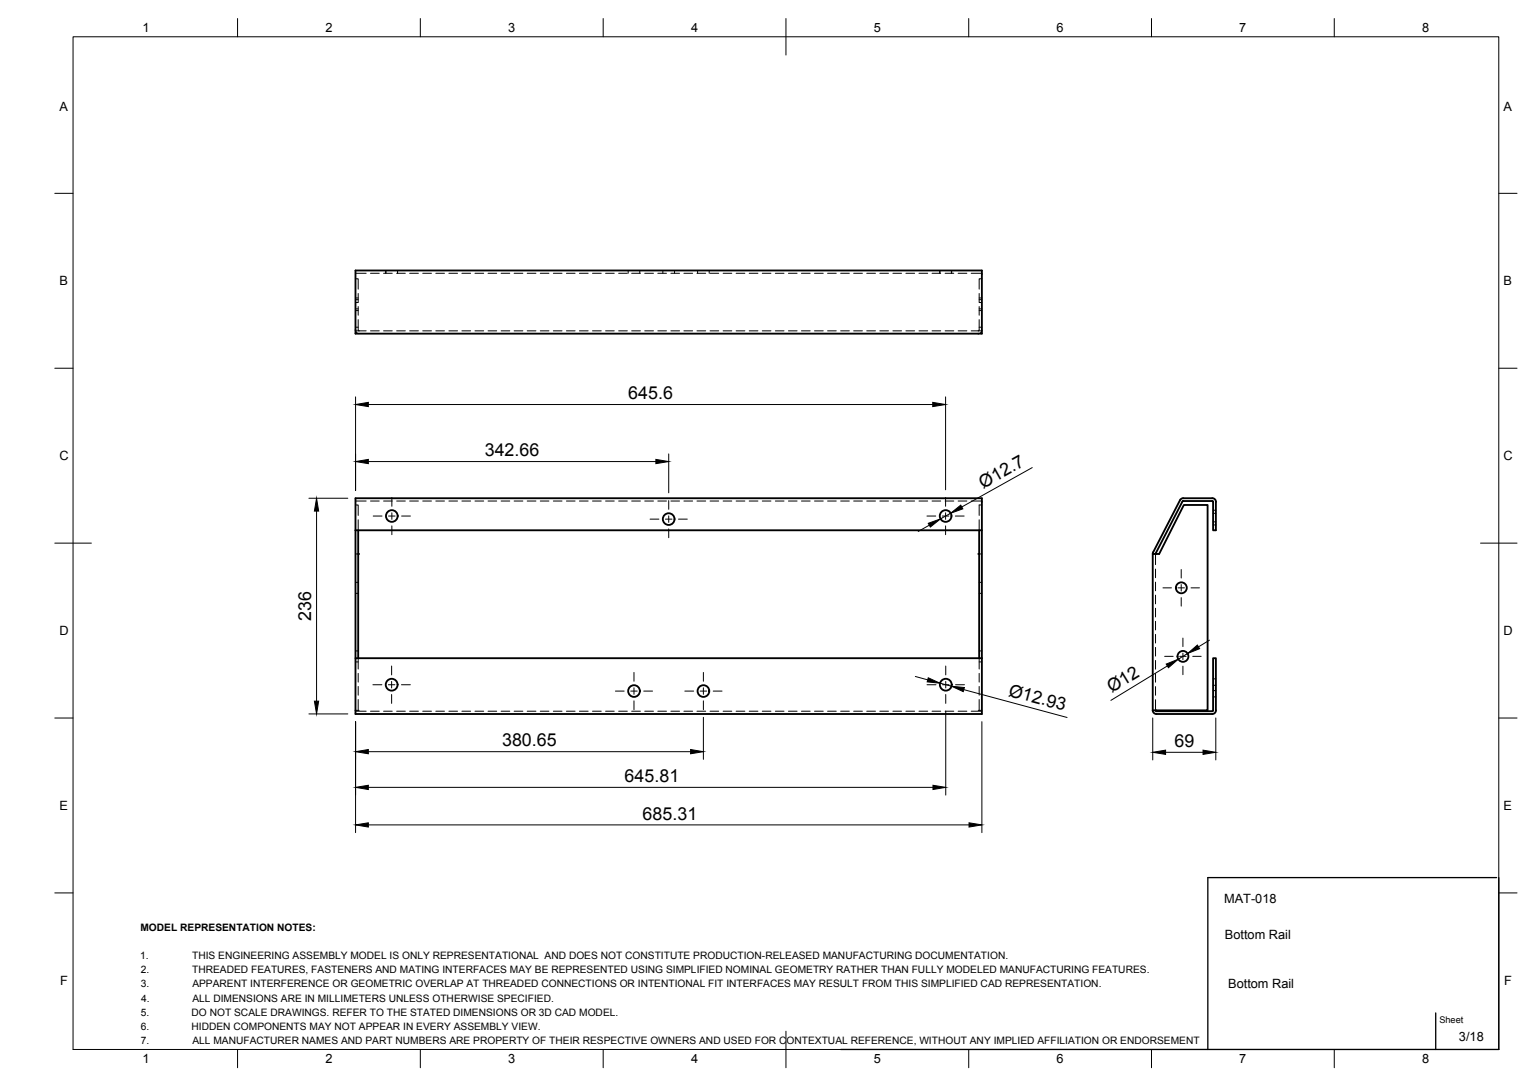
ISO-10303-21;
HEADER;
/* Generated by software containing ST-Developer
 * from STEP Tools, Inc. (www.steptools.com) 
 */

FILE_DESCRIPTION(
/* description */ ('STEP AP214'),
/* implementation_level */ '2;1');

FILE_NAME(
/* name */ 'Bottom Rail.step',
/* time_stamp */ '2026-11-14T06:16:09-08:00',
/* author */ (''),
/* organization */ (''),
/* preprocessor_version */ 'ST-DEVELOPER v20.2',
/* originating_system */ 'Autodesk Translation Framework v15.17.0.0',
/* authorisation */ '');

FILE_SCHEMA (('AUTOMOTIVE_DESIGN { 1 0 10303 214 3 1 1 }'));
ENDSEC;

DATA;
#10=MECHANICAL_DESIGN_GEOMETRIC_PRESENTATION_REPRESENTATION('',(#347),#18006);
#315=SHAPE_REPRESENTATION_RELATIONSHIP('SRR','None',#18071,#331);
#331=ADVANCED_BREP_SHAPE_REPRESENTATION('',(#363),#17988);
#347=STYLED_ITEM('',(#18170),#363);
#363=MANIFOLD_SOLID_BREP('Body1',#9556);
#379=FACE_BOUND('',#1453,.T.);
#380=FACE_BOUND('',#1454,.T.);
#381=FACE_BOUND('',#1455,.T.);
#382=FACE_BOUND('',#1456,.T.);
#383=FACE_BOUND('',#1459,.T.);
#384=FACE_BOUND('',#1460,.T.);
#385=FACE_BOUND('',#1461,.T.);
#386=FACE_BOUND('',#1462,.T.);
#387=FACE_BOUND('',#1472,.T.);
#388=FACE_BOUND('',#1473,.T.);
#389=FACE_BOUND('',#1474,.T.);
#390=FACE_BOUND('',#1477,.T.);
#391=FACE_BOUND('',#1478,.T.);
#392=FACE_BOUND('',#1479,.T.);
#393=FACE_BOUND('',#1497,.T.);
#394=FACE_BOUND('',#1498,.T.);
#395=FACE_BOUND('',#1500,.T.);
#396=FACE_BOUND('',#1501,.T.);
#397=FACE_BOUND('',#1512,.T.);
#398=FACE_BOUND('',#1513,.T.);
#399=FACE_BOUND('',#1515,.T.);
#400=FACE_BOUND('',#1516,.T.);
#502=PLANE('',#9784);
#503=PLANE('',#9786);
#504=PLANE('',#9788);
#505=PLANE('',#9789);
#506=PLANE('',#9790);
#507=PLANE('',#9792);
#508=PLANE('',#9794);
#509=PLANE('',#9797);
#510=PLANE('',#9798);
#511=PLANE('',#9801);
#512=PLANE('',#9802);
#513=PLANE('',#9805);
#514=PLANE('',#9806);
#515=PLANE('',#9809);
#516=PLANE('',#9810);
#517=PLANE('',#9813);
#518=PLANE('',#9816);
#519=PLANE('',#9817);
#520=PLANE('',#9820);
#521=PLANE('',#9821);
#522=PLANE('',#9824);
#523=PLANE('',#9827);
#524=PLANE('',#9828);
#525=PLANE('',#9831);
#526=PLANE('',#9832);
#527=PLANE('',#9833);
#528=PLANE('',#9834);
#529=PLANE('',#9836);
#530=PLANE('',#9839);
#531=PLANE('',#9841);
#532=PLANE('',#9843);
#533=PLANE('',#9844);
#534=PLANE('',#9845);
#535=PLANE('',#9847);
#536=PLANE('',#9849);
#537=PLANE('',#9852);
#538=PLANE('',#9854);
#539=PLANE('',#9855);
#540=PLANE('',#9856);
#541=PLANE('',#9859);
#542=PLANE('',#9864);
#543=PLANE('',#9865);
#544=PLANE('',#9866);
#545=PLANE('',#9867);
#546=PLANE('',#9868);
#547=PLANE('',#9869);
#548=PLANE('',#9870);
#549=PLANE('',#9871);
#550=PLANE('',#9874);
#551=PLANE('',#9879);
#552=PLANE('',#9880);
#553=PLANE('',#9881);
#554=PLANE('',#9882);
#555=PLANE('',#9883);
#556=PLANE('',#9884);
#557=PLANE('',#9885);
#841=FACE_OUTER_BOUND('',#1417,.T.);
#842=FACE_OUTER_BOUND('',#1418,.T.);
#843=FACE_OUTER_BOUND('',#1419,.T.);
#844=FACE_OUTER_BOUND('',#1420,.T.);
#845=FACE_OUTER_BOUND('',#1421,.T.);
#846=FACE_OUTER_BOUND('',#1422,.T.);
#847=FACE_OUTER_BOUND('',#1423,.T.);
#848=FACE_OUTER_BOUND('',#1424,.T.);
#849=FACE_OUTER_BOUND('',#1425,.T.);
#850=FACE_OUTER_BOUND('',#1426,.T.);
#851=FACE_OUTER_BOUND('',#1427,.T.);
#852=FACE_OUTER_BOUND('',#1428,.T.);
#853=FACE_OUTER_BOUND('',#1429,.T.);
#854=FACE_OUTER_BOUND('',#1430,.T.);
#855=FACE_OUTER_BOUND('',#1431,.T.);
#856=FACE_OUTER_BOUND('',#1432,.T.);
#857=FACE_OUTER_BOUND('',#1433,.T.);
#858=FACE_OUTER_BOUND('',#1434,.T.);
#859=FACE_OUTER_BOUND('',#1435,.T.);
#860=FACE_OUTER_BOUND('',#1436,.T.);
#861=FACE_OUTER_BOUND('',#1437,.T.);
#862=FACE_OUTER_BOUND('',#1438,.T.);
#863=FACE_OUTER_BOUND('',#1439,.T.);
#864=FACE_OUTER_BOUND('',#1440,.T.);
#865=FACE_OUTER_BOUND('',#1441,.T.);
#866=FACE_OUTER_BOUND('',#1442,.T.);
#867=FACE_OUTER_BOUND('',#1443,.T.);
#868=FACE_OUTER_BOUND('',#1444,.T.);
#869=FACE_OUTER_BOUND('',#1445,.T.);
#870=FACE_OUTER_BOUND('',#1446,.T.);
#871=FACE_OUTER_BOUND('',#1447,.T.);
#872=FACE_OUTER_BOUND('',#1448,.T.);
#873=FACE_OUTER_BOUND('',#1449,.T.);
#874=FACE_OUTER_BOUND('',#1450,.T.);
#875=FACE_OUTER_BOUND('',#1451,.T.);
#876=FACE_OUTER_BOUND('',#1452,.T.);
#877=FACE_OUTER_BOUND('',#1457,.T.);
#878=FACE_OUTER_BOUND('',#1458,.T.);
#879=FACE_OUTER_BOUND('',#1463,.T.);
#880=FACE_OUTER_BOUND('',#1464,.T.);
#881=FACE_OUTER_BOUND('',#1465,.T.);
#882=FACE_OUTER_BOUND('',#1466,.T.);
#883=FACE_OUTER_BOUND('',#1467,.T.);
#884=FACE_OUTER_BOUND('',#1468,.T.);
#885=FACE_OUTER_BOUND('',#1469,.T.);
#886=FACE_OUTER_BOUND('',#1470,.T.);
#887=FACE_OUTER_BOUND('',#1471,.T.);
#888=FACE_OUTER_BOUND('',#1475,.T.);
#889=FACE_OUTER_BOUND('',#1476,.T.);
#890=FACE_OUTER_BOUND('',#1480,.T.);
#891=FACE_OUTER_BOUND('',#1481,.T.);
#892=FACE_OUTER_BOUND('',#1482,.T.);
#893=FACE_OUTER_BOUND('',#1483,.T.);
#894=FACE_OUTER_BOUND('',#1484,.T.);
#895=FACE_OUTER_BOUND('',#1485,.T.);
#896=FACE_OUTER_BOUND('',#1486,.T.);
#897=FACE_OUTER_BOUND('',#1487,.T.);
#898=FACE_OUTER_BOUND('',#1488,.T.);
#899=FACE_OUTER_BOUND('',#1489,.T.);
#900=FACE_OUTER_BOUND('',#1490,.T.);
#901=FACE_OUTER_BOUND('',#1491,.T.);
#902=FACE_OUTER_BOUND('',#1492,.T.);
#903=FACE_OUTER_BOUND('',#1493,.T.);
#904=FACE_OUTER_BOUND('',#1494,.T.);
#905=FACE_OUTER_BOUND('',#1495,.T.);
#906=FACE_OUTER_BOUND('',#1496,.T.);
#907=FACE_OUTER_BOUND('',#1499,.T.);
#908=FACE_OUTER_BOUND('',#1502,.T.);
#909=FACE_OUTER_BOUND('',#1503,.T.);
#910=FACE_OUTER_BOUND('',#1504,.T.);
#911=FACE_OUTER_BOUND('',#1505,.T.);
#912=FACE_OUTER_BOUND('',#1506,.T.);
#913=FACE_OUTER_BOUND('',#1507,.T.);
#914=FACE_OUTER_BOUND('',#1508,.T.);
#915=FACE_OUTER_BOUND('',#1509,.T.);
#916=FACE_OUTER_BOUND('',#1510,.T.);
#917=FACE_OUTER_BOUND('',#1511,.T.);
#918=FACE_OUTER_BOUND('',#1514,.T.);
#919=FACE_OUTER_BOUND('',#1517,.T.);
#920=FACE_OUTER_BOUND('',#1518,.T.);
#921=FACE_OUTER_BOUND('',#1519,.T.);
#1417=EDGE_LOOP('',(#6152,#6153,#6154,#6155));
#1418=EDGE_LOOP('',(#6156,#6157,#6158,#6159));
#1419=EDGE_LOOP('',(#6160,#6161,#6162,#6163));
#1420=EDGE_LOOP('',(#6164,#6165,#6166,#6167));
#1421=EDGE_LOOP('',(#6168,#6169,#6170,#6171));
#1422=EDGE_LOOP('',(#6172,#6173,#6174,#6175));
#1423=EDGE_LOOP('',(#6176,#6177,#6178,#6179));
#1424=EDGE_LOOP('',(#6180,#6181,#6182,#6183));
#1425=EDGE_LOOP('',(#6184,#6185,#6186,#6187));
#1426=EDGE_LOOP('',(#6188,#6189,#6190,#6191));
#1427=EDGE_LOOP('',(#6192,#6193,#6194,#6195));
#1428=EDGE_LOOP('',(#6196,#6197,#6198,#6199));
#1429=EDGE_LOOP('',(#6200,#6201,#6202,#6203));
#1430=EDGE_LOOP('',(#6204,#6205,#6206,#6207));
#1431=EDGE_LOOP('',(#6208,#6209,#6210,#6211));
#1432=EDGE_LOOP('',(#6212,#6213,#6214,#6215));
#1433=EDGE_LOOP('',(#6216,#6217,#6218,#6219));
#1434=EDGE_LOOP('',(#6220,#6221,#6222,#6223));
#1435=EDGE_LOOP('',(#6224,#6225,#6226,#6227));
#1436=EDGE_LOOP('',(#6228,#6229,#6230,#6231));
#1437=EDGE_LOOP('',(#6232,#6233,#6234,#6235));
#1438=EDGE_LOOP('',(#6236,#6237,#6238,#6239));
#1439=EDGE_LOOP('',(#6240,#6241,#6242,#6243));
#1440=EDGE_LOOP('',(#6244,#6245,#6246,#6247));
#1441=EDGE_LOOP('',(#6248,#6249,#6250,#6251));
#1442=EDGE_LOOP('',(#6252,#6253,#6254,#6255));
#1443=EDGE_LOOP('',(#6256,#6257,#6258,#6259));
#1444=EDGE_LOOP('',(#6260,#6261,#6262,#6263));
#1445=EDGE_LOOP('',(#6264,#6265,#6266,#6267));
#1446=EDGE_LOOP('',(#6268,#6269,#6270,#6271));
#1447=EDGE_LOOP('',(#6272,#6273,#6274,#6275));
#1448=EDGE_LOOP('',(#6276,#6277,#6278,#6279));
#1449=EDGE_LOOP('',(#6280,#6281,#6282,#6283));
#1450=EDGE_LOOP('',(#6284,#6285,#6286,#6287));
#1451=EDGE_LOOP('',(#6288,#6289,#6290,#6291));
#1452=EDGE_LOOP('',(#6292,#6293,#6294,#6295));
#1453=EDGE_LOOP('',(#6296));
#1454=EDGE_LOOP('',(#6297));
#1455=EDGE_LOOP('',(#6298));
#1456=EDGE_LOOP('',(#6299));
#1457=EDGE_LOOP('',(#6300,#6301,#6302,#6303));
#1458=EDGE_LOOP('',(#6304,#6305,#6306,#6307));
#1459=EDGE_LOOP('',(#6308));
#1460=EDGE_LOOP('',(#6309));
#1461=EDGE_LOOP('',(#6310));
#1462=EDGE_LOOP('',(#6311));
#1463=EDGE_LOOP('',(#6312,#6313,#6314,#6315));
#1464=EDGE_LOOP('',(#6316,#6317,#6318,#6319));
#1465=EDGE_LOOP('',(#6320,#6321,#6322,#6323,#6324,#6325));
#1466=EDGE_LOOP('',(#6326,#6327,#6328,#6329,#6330,#6331));
#1467=EDGE_LOOP('',(#6332,#6333,#6334,#6335));
#1468=EDGE_LOOP('',(#6336,#6337,#6338,#6339));
#1469=EDGE_LOOP('',(#6340,#6341,#6342,#6343));
#1470=EDGE_LOOP('',(#6344,#6345,#6346,#6347));
#1471=EDGE_LOOP('',(#6348,#6349,#6350,#6351));
#1472=EDGE_LOOP('',(#6352));
#1473=EDGE_LOOP('',(#6353));
#1474=EDGE_LOOP('',(#6354));
#1475=EDGE_LOOP('',(#6355,#6356,#6357,#6358));
#1476=EDGE_LOOP('',(#6359,#6360,#6361,#6362));
#1477=EDGE_LOOP('',(#6363));
#1478=EDGE_LOOP('',(#6364));
#1479=EDGE_LOOP('',(#6365));
#1480=EDGE_LOOP('',(#6366,#6367,#6368,#6369));
#1481=EDGE_LOOP('',(#6370,#6371,#6372,#6373));
#1482=EDGE_LOOP('',(#6374,#6375,#6376,#6377));
#1483=EDGE_LOOP('',(#6378,#6379,#6380,#6381));
#1484=EDGE_LOOP('',(#6382,#6383,#6384,#6385,#6386,#6387,#6388,#6389));
#1485=EDGE_LOOP('',(#6390,#6391,#6392,#6393,#6394,#6395,#6396,#6397));
#1486=EDGE_LOOP('',(#6398,#6399,#6400,#6401));
#1487=EDGE_LOOP('',(#6402,#6403,#6404,#6405));
#1488=EDGE_LOOP('',(#6406,#6407,#6408,#6409));
#1489=EDGE_LOOP('',(#6410,#6411,#6412,#6413));
#1490=EDGE_LOOP('',(#6414,#6415,#6416,#6417));
#1491=EDGE_LOOP('',(#6418,#6419,#6420,#6421));
#1492=EDGE_LOOP('',(#6422,#6423,#6424,#6425,#6426,#6427));
#1493=EDGE_LOOP('',(#6428,#6429,#6430,#6431));
#1494=EDGE_LOOP('',(#6432,#6433,#6434,#6435));
#1495=EDGE_LOOP('',(#6436,#6437,#6438,#6439));
#1496=EDGE_LOOP('',(#6440,#6441,#6442,#6443,#6444,#6445));
#1497=EDGE_LOOP('',(#6446));
#1498=EDGE_LOOP('',(#6447));
#1499=EDGE_LOOP('',(#6448,#6449,#6450,#6451,#6452,#6453));
#1500=EDGE_LOOP('',(#6454));
#1501=EDGE_LOOP('',(#6455));
#1502=EDGE_LOOP('',(#6456,#6457,#6458,#6459));
#1503=EDGE_LOOP('',(#6460,#6461,#6462,#6463));
#1504=EDGE_LOOP('',(#6464,#6465,#6466,#6467));
#1505=EDGE_LOOP('',(#6468,#6469,#6470,#6471));
#1506=EDGE_LOOP('',(#6472,#6473,#6474,#6475));
#1507=EDGE_LOOP('',(#6476,#6477,#6478,#6479,#6480,#6481));
#1508=EDGE_LOOP('',(#6482,#6483,#6484,#6485));
#1509=EDGE_LOOP('',(#6486,#6487,#6488,#6489));
#1510=EDGE_LOOP('',(#6490,#6491,#6492,#6493));
#1511=EDGE_LOOP('',(#6494,#6495,#6496,#6497,#6498,#6499));
#1512=EDGE_LOOP('',(#6500));
#1513=EDGE_LOOP('',(#6501));
#1514=EDGE_LOOP('',(#6502,#6503,#6504,#6505,#6506,#6507));
#1515=EDGE_LOOP('',(#6508));
#1516=EDGE_LOOP('',(#6509));
#1517=EDGE_LOOP('',(#6510,#6511,#6512,#6513));
#1518=EDGE_LOOP('',(#6514,#6515,#6516,#6517));
#1519=EDGE_LOOP('',(#6518,#6519,#6520,#6521));
#2116=LINE('',#13815,#2840);
#2117=LINE('',#13821,#2841);
#2118=LINE('',#13827,#2842);
#2119=LINE('',#13833,#2843);
#2120=LINE('',#13839,#2844);
#2121=LINE('',#13845,#2845);
#2122=LINE('',#13851,#2846);
#2123=LINE('',#13857,#2847);
#2124=LINE('',#13863,#2848);
#2125=LINE('',#13869,#2849);
#2126=LINE('',#13875,#2850);
#2127=LINE('',#13880,#2851);
#2128=LINE('',#13884,#2852);
#2129=LINE('',#13885,#2853);
#2130=LINE('',#13889,#2854);
#2131=LINE('',#13893,#2855);
#2132=LINE('',#13894,#2856);
#2133=LINE('',#13897,#2857);
#2134=LINE('',#13898,#2858);
#2135=LINE('',#13900,#2859);
#2136=LINE('',#13901,#2860);
#2137=LINE('',#13905,#2861);
#2138=LINE('',#13907,#2862);
#2139=LINE('',#13909,#2863);
#2140=LINE('',#13910,#2864);
#2141=LINE('',#13914,#2865);
#2142=LINE('',#13917,#2866);
#2143=LINE('',#13918,#2867);
#2144=LINE('',#13921,#2868);
#2145=LINE('',#13925,#2869);
#2146=LINE('',#13926,#2870);
#2147=LINE('',#13930,#2871);
#2148=LINE('',#13934,#2872);
#2149=LINE('',#13938,#2873);
#2150=LINE('',#13940,#2874);
#2151=LINE('',#13941,#2875);
#2152=LINE('',#13945,#2876);
#2153=LINE('',#13949,#2877);
#2154=LINE('',#13953,#2878);
#2155=LINE('',#13955,#2879);
#2156=LINE('',#13956,#2880);
#2157=LINE('',#13960,#2881);
#2158=LINE('',#13965,#2882);
#2159=LINE('',#13967,#2883);
#2160=LINE('',#13968,#2884);
#2161=LINE('',#13972,#2885);
#2162=LINE('',#13976,#2886);
#2163=LINE('',#13979,#2887);
#2164=LINE('',#13980,#2888);
#2165=LINE('',#13987,#2889);
#2166=LINE('',#13991,#2890);
#2167=LINE('',#13992,#2891);
#2168=LINE('',#13996,#2892);
#2169=LINE('',#14001,#2893);
#2170=LINE('',#14003,#2894);
#2171=LINE('',#14004,#2895);
#2172=LINE('',#14009,#2896);
#2173=LINE('',#14014,#2897);
#2174=LINE('',#14019,#2898);
#2175=LINE('',#14021,#2899);
#2176=LINE('',#14022,#2900);
#2177=LINE('',#14026,#2901);
#2178=LINE('',#14030,#2902);
#2179=LINE('',#14033,#2903);
#2180=LINE('',#14034,#2904);
#2181=LINE('',#14037,#2905);
#2182=LINE('',#14038,#2906);
#2183=LINE('',#14039,#2907);
#2184=LINE('',#14042,#2908);
#2185=LINE('',#14043,#2909);
#2186=LINE('',#14045,#2910);
#2187=LINE('',#14046,#2911);
#2188=LINE('',#14048,#2912);
#2189=LINE('',#14050,#2913);
#2190=LINE('',#14053,#2914);
#2191=LINE('',#14055,#2915);
#2192=LINE('',#14057,#2916);
#2193=LINE('',#14059,#2917);
#2194=LINE('',#14061,#2918);
#2195=LINE('',#14064,#2919);
#2196=LINE('',#14065,#2920);
#2197=LINE('',#14068,#2921);
#2198=LINE('',#14069,#2922);
#2199=LINE('',#14071,#2923);
#2200=LINE('',#14072,#2924);
#2201=LINE('',#14074,#2925);
#2202=LINE('',#14076,#2926);
#2203=LINE('',#14078,#2927);
#2204=LINE('',#14080,#2928);
#2205=LINE('',#14082,#2929);
#2206=LINE('',#14083,#2930);
#2207=LINE('',#14085,#2931);
#2208=LINE('',#14086,#2932);
#2209=LINE('',#14087,#2933);
#2210=LINE('',#14089,#2934);
#2211=LINE('',#14097,#2935);
#2212=LINE('',#14104,#2936);
#2213=LINE('',#14106,#2937);
#2214=LINE('',#14108,#2938);
#2215=LINE('',#14111,#2939);
#2216=LINE('',#14113,#2940);
#2217=LINE('',#14114,#2941);
#2218=LINE('',#14117,#2942);
#2219=LINE('',#14119,#2943);
#2220=LINE('',#14120,#2944);
#2221=LINE('',#14123,#2945);
#2222=LINE('',#14125,#2946);
#2223=LINE('',#14126,#2947);
#2224=LINE('',#14129,#2948);
#2225=LINE('',#14131,#2949);
#2226=LINE('',#14132,#2950);
#2227=LINE('',#14134,#2951);
#2228=LINE('',#14136,#2952);
#2229=LINE('',#14143,#2953);
#2230=LINE('',#14149,#2954);
#2231=LINE('',#14151,#2955);
#2232=LINE('',#14153,#2956);
#2233=LINE('',#14156,#2957);
#2234=LINE('',#14158,#2958);
#2235=LINE('',#14159,#2959);
#2236=LINE('',#14162,#2960);
#2237=LINE('',#14164,#2961);
#2238=LINE('',#14165,#2962);
#2239=LINE('',#14168,#2963);
#2240=LINE('',#14170,#2964);
#2241=LINE('',#14171,#2965);
#2242=LINE('',#14174,#2966);
#2243=LINE('',#14176,#2967);
#2244=LINE('',#14177,#2968);
#2245=LINE('',#14179,#2969);
#2246=LINE('',#14181,#2970);
#2840=VECTOR('',#10869,6.00000000000002);
#2841=VECTOR('',#10876,6.00000000000001);
#2842=VECTOR('',#10883,6.00000000000002);
#2843=VECTOR('',#10890,6.00000000000001);
#2844=VECTOR('',#10897,6.34999999999999);
#2845=VECTOR('',#10904,6.35000000000122);
#2846=VECTOR('',#10911,6.35000000000122);
#2847=VECTOR('',#10918,6.46290152238551);
#2848=VECTOR('',#10925,6.4629015223855);
#2849=VECTOR('',#10932,6.34999999999994);
#2850=VECTOR('',#10939,6.34999999999994);
#2851=VECTOR('',#10944,1000.);
#2852=VECTOR('',#10947,1000.);
#2853=VECTOR('',#10948,1000.);
#2854=VECTOR('',#10951,1000.);
#2855=VECTOR('',#10954,1000.);
#2856=VECTOR('',#10955,1000.);
#2857=VECTOR('',#10958,1000.);
#2858=VECTOR('',#10959,1000.);
#2859=VECTOR('',#10960,1000.);
#2860=VECTOR('',#10961,1000.);
#2861=VECTOR('',#10964,1000.);
#2862=VECTOR('',#10965,1000.);
#2863=VECTOR('',#10966,1000.);
#2864=VECTOR('',#10967,1000.);
#2865=VECTOR('',#10970,1000.);
#2866=VECTOR('',#10973,1000.);
#2867=VECTOR('',#10974,1000.);
#2868=VECTOR('',#10977,1000.);
#2869=VECTOR('',#10980,1000.);
#2870=VECTOR('',#10981,1000.);
#2871=VECTOR('',#10984,1000.);
#2872=VECTOR('',#10987,1000.);
#2873=VECTOR('',#10992,1000.);
#2874=VECTOR('',#10993,1000.);
#2875=VECTOR('',#10994,1000.);
#2876=VECTOR('',#10997,1000.);
#2877=VECTOR('',#11000,1000.);
#2878=VECTOR('',#11005,1000.);
#2879=VECTOR('',#11006,1000.);
#2880=VECTOR('',#11007,1000.);
#2881=VECTOR('',#11010,1000.);
#2882=VECTOR('',#11017,1000.);
#2883=VECTOR('',#11018,1000.);
#2884=VECTOR('',#11019,1000.);
#2885=VECTOR('',#11022,1000.);
#2886=VECTOR('',#11025,1000.);
#2887=VECTOR('',#11030,1000.);
#2888=VECTOR('',#11031,1000.);
#2889=VECTOR('',#11040,1000.);
#2890=VECTOR('',#11047,1000.);
#2891=VECTOR('',#11048,1000.);
#2892=VECTOR('',#11051,1000.);
#2893=VECTOR('',#11058,1000.);
#2894=VECTOR('',#11059,1000.);
#2895=VECTOR('',#11060,1000.);
#2896=VECTOR('',#11065,1000.);
#2897=VECTOR('',#11070,1000.);
#2898=VECTOR('',#11077,1000.);
#2899=VECTOR('',#11078,1000.);
#2900=VECTOR('',#11079,1000.);
#2901=VECTOR('',#11082,1000.);
#2902=VECTOR('',#11085,1000.);
#2903=VECTOR('',#11090,1000.);
#2904=VECTOR('',#11091,1000.);
#2905=VECTOR('',#11094,1000.);
#2906=VECTOR('',#11095,1000.);
#2907=VECTOR('',#11096,1000.);
#2908=VECTOR('',#11099,1000.);
#2909=VECTOR('',#11100,1000.);
#2910=VECTOR('',#11103,1000.);
#2911=VECTOR('',#11104,1000.);
#2912=VECTOR('',#11107,1000.);
#2913=VECTOR('',#11110,1000.);
#2914=VECTOR('',#11115,1000.);
#2915=VECTOR('',#11118,1000.);
#2916=VECTOR('',#11121,1000.);
#2917=VECTOR('',#11124,1000.);
#2918=VECTOR('',#11127,1000.);
#2919=VECTOR('',#11130,1000.);
#2920=VECTOR('',#11131,1000.);
#2921=VECTOR('',#11134,1000.);
#2922=VECTOR('',#11135,1000.);
#2923=VECTOR('',#11138,1000.);
#2924=VECTOR('',#11139,1000.);
#2925=VECTOR('',#11142,1000.);
#2926=VECTOR('',#11145,1000.);
#2927=VECTOR('',#11148,1000.);
#2928=VECTOR('',#11151,1000.);
#2929=VECTOR('',#11154,1000.);
#2930=VECTOR('',#11155,1000.);
#2931=VECTOR('',#11158,1000.);
#2932=VECTOR('',#11159,1000.);
#2933=VECTOR('',#11160,1000.);
#2934=VECTOR('',#11163,1000.);
#2935=VECTOR('',#11174,1000.);
#2936=VECTOR('',#11183,1000.);
#2937=VECTOR('',#11186,1000.);
#2938=VECTOR('',#11189,1000.);
#2939=VECTOR('',#11192,1000.);
#2940=VECTOR('',#11193,1000.);
#2941=VECTOR('',#11194,1000.);
#2942=VECTOR('',#11197,1000.);
#2943=VECTOR('',#11198,1000.);
#2944=VECTOR('',#11199,1000.);
#2945=VECTOR('',#11202,1000.);
#2946=VECTOR('',#11203,1000.);
#2947=VECTOR('',#11204,1000.);
#2948=VECTOR('',#11207,1000.);
#2949=VECTOR('',#11208,1000.);
#2950=VECTOR('',#11209,1000.);
#2951=VECTOR('',#11212,1000.);
#2952=VECTOR('',#11215,1000.);
#2953=VECTOR('',#11224,1000.);
#2954=VECTOR('',#11231,1000.);
#2955=VECTOR('',#11234,1000.);
#2956=VECTOR('',#11237,1000.);
#2957=VECTOR('',#11240,1000.);
#2958=VECTOR('',#11241,1000.);
#2959=VECTOR('',#11242,1000.);
#2960=VECTOR('',#11245,1000.);
#2961=VECTOR('',#11246,1000.);
#2962=VECTOR('',#11247,1000.);
#2963=VECTOR('',#11250,1000.);
#2964=VECTOR('',#11251,1000.);
#2965=VECTOR('',#11252,1000.);
#2966=VECTOR('',#11255,1000.);
#2967=VECTOR('',#11256,1000.);
#2968=VECTOR('',#11257,1000.);
#2969=VECTOR('',#11260,1000.);
#2970=VECTOR('',#11263,1000.);
#3564=CIRCLE('',#9752,6.00000000000002);
#3565=CIRCLE('',#9753,6.00000000000002);
#3566=CIRCLE('',#9755,6.00000000000001);
#3567=CIRCLE('',#9756,6.00000000000001);
#3568=CIRCLE('',#9758,6.00000000000002);
#3569=CIRCLE('',#9759,6.00000000000002);
#3570=CIRCLE('',#9761,6.00000000000001);
#3571=CIRCLE('',#9762,6.00000000000001);
#3572=CIRCLE('',#9764,6.34999999999999);
#3573=CIRCLE('',#9765,6.34999999999999);
#3574=CIRCLE('',#9767,6.35000000000122);
#3575=CIRCLE('',#9768,6.35000000000122);
#3576=CIRCLE('',#9770,6.35000000000122);
#3577=CIRCLE('',#9771,6.35000000000122);
#3578=CIRCLE('',#9773,6.46290152238551);
#3579=CIRCLE('',#9774,6.4629015223855);
#3580=CIRCLE('',#9776,6.4629015223855);
#3581=CIRCLE('',#9777,6.4629015223855);
#3582=CIRCLE('',#9779,6.34999999999994);
#3583=CIRCLE('',#9780,6.34999999999994);
#3584=CIRCLE('',#9782,6.34999999999994);
#3585=CIRCLE('',#9783,6.34999999999994);
#3586=CIRCLE('',#9785,4.);
#3587=CIRCLE('',#9787,4.);
#3588=CIRCLE('',#9791,4.);
#3589=CIRCLE('',#9793,4.);
#3590=CIRCLE('',#9795,4.);
#3591=CIRCLE('',#9796,1.);
#3592=CIRCLE('',#9799,4.);
#3593=CIRCLE('',#9800,1.);
#3594=CIRCLE('',#9803,4.);
#3595=CIRCLE('',#9804,1.);
#3596=CIRCLE('',#9807,4.);
#3597=CIRCLE('',#9808,1.);
#3598=CIRCLE('',#9811,4.);
#3599=CIRCLE('',#9812,1.);
#3600=CIRCLE('',#9814,4.);
#3601=CIRCLE('',#9815,1.);
#3602=CIRCLE('',#9818,4.);
#3603=CIRCLE('',#9819,1.);
#3604=CIRCLE('',#9822,4.);
#3605=CIRCLE('',#9823,1.);
#3606=CIRCLE('',#9825,4.);
#3607=CIRCLE('',#9826,1.);
#3608=CIRCLE('',#9829,4.);
#3609=CIRCLE('',#9830,1.);
#3610=CIRCLE('',#9857,4.);
#3611=CIRCLE('',#9858,1.);
#3612=CIRCLE('',#9860,4.);
#3613=CIRCLE('',#9861,1.);
#3614=CIRCLE('',#9872,1.);
#3615=CIRCLE('',#9873,4.);
#3616=CIRCLE('',#9875,4.);
#3617=CIRCLE('',#9876,1.);
#4013=VERTEX_POINT('',#13812);
#4014=VERTEX_POINT('',#13814);
#4015=VERTEX_POINT('',#13818);
#4016=VERTEX_POINT('',#13820);
#4017=VERTEX_POINT('',#13824);
#4018=VERTEX_POINT('',#13826);
#4019=VERTEX_POINT('',#13830);
#4020=VERTEX_POINT('',#13832);
#4021=VERTEX_POINT('',#13836);
#4022=VERTEX_POINT('',#13838);
#4023=VERTEX_POINT('',#13842);
#4024=VERTEX_POINT('',#13844);
#4025=VERTEX_POINT('',#13848);
#4026=VERTEX_POINT('',#13850);
#4027=VERTEX_POINT('',#13854);
#4028=VERTEX_POINT('',#13856);
#4029=VERTEX_POINT('',#13860);
#4030=VERTEX_POINT('',#13862);
#4031=VERTEX_POINT('',#13866);
#4032=VERTEX_POINT('',#13868);
#4033=VERTEX_POINT('',#13872);
#4034=VERTEX_POINT('',#13874);
#4035=VERTEX_POINT('',#13878);
#4036=VERTEX_POINT('',#13879);
#4037=VERTEX_POINT('',#13881);
#4038=VERTEX_POINT('',#13883);
#4039=VERTEX_POINT('',#13887);
#4040=VERTEX_POINT('',#13888);
#4041=VERTEX_POINT('',#13890);
#4042=VERTEX_POINT('',#13892);
#4043=VERTEX_POINT('',#13896);
#4044=VERTEX_POINT('',#13899);
#4045=VERTEX_POINT('',#13903);
#4046=VERTEX_POINT('',#13904);
#4047=VERTEX_POINT('',#13906);
#4048=VERTEX_POINT('',#13908);
#4049=VERTEX_POINT('',#13912);
#4050=VERTEX_POINT('',#13913);
#4051=VERTEX_POINT('',#13916);
#4052=VERTEX_POINT('',#13920);
#4053=VERTEX_POINT('',#13922);
#4054=VERTEX_POINT('',#13924);
#4055=VERTEX_POINT('',#13928);
#4056=VERTEX_POINT('',#13929);
#4057=VERTEX_POINT('',#13931);
#4058=VERTEX_POINT('',#13933);
#4059=VERTEX_POINT('',#13937);
#4060=VERTEX_POINT('',#13939);
#4061=VERTEX_POINT('',#13943);
#4062=VERTEX_POINT('',#13944);
#4063=VERTEX_POINT('',#13946);
#4064=VERTEX_POINT('',#13948);
#4065=VERTEX_POINT('',#13952);
#4066=VERTEX_POINT('',#13954);
#4067=VERTEX_POINT('',#13958);
#4068=VERTEX_POINT('',#13959);
#4069=VERTEX_POINT('',#13964);
#4070=VERTEX_POINT('',#13966);
#4071=VERTEX_POINT('',#13970);
#4072=VERTEX_POINT('',#13971);
#4073=VERTEX_POINT('',#13973);
#4074=VERTEX_POINT('',#13975);
#4075=VERTEX_POINT('',#13985);
#4076=VERTEX_POINT('',#13986);
#4077=VERTEX_POINT('',#13994);
#4078=VERTEX_POINT('',#13995);
#4079=VERTEX_POINT('',#14000);
#4080=VERTEX_POINT('',#14002);
#4081=VERTEX_POINT('',#14006);
#4082=VERTEX_POINT('',#14008);
#4083=VERTEX_POINT('',#14012);
#4084=VERTEX_POINT('',#14013);
#4085=VERTEX_POINT('',#14018);
#4086=VERTEX_POINT('',#14020);
#4087=VERTEX_POINT('',#14024);
#4088=VERTEX_POINT('',#14025);
#4089=VERTEX_POINT('',#14027);
#4090=VERTEX_POINT('',#14029);
#4091=VERTEX_POINT('',#14036);
#4092=VERTEX_POINT('',#14041);
#4093=VERTEX_POINT('',#14063);
#4094=VERTEX_POINT('',#14067);
#4095=VERTEX_POINT('',#14094);
#4096=VERTEX_POINT('',#14096);
#4097=VERTEX_POINT('',#14100);
#4098=VERTEX_POINT('',#14102);
#4099=VERTEX_POINT('',#14110);
#4100=VERTEX_POINT('',#14112);
#4101=VERTEX_POINT('',#14116);
#4102=VERTEX_POINT('',#14118);
#4103=VERTEX_POINT('',#14122);
#4104=VERTEX_POINT('',#14124);
#4105=VERTEX_POINT('',#14128);
#4106=VERTEX_POINT('',#14130);
#4107=VERTEX_POINT('',#14139);
#4108=VERTEX_POINT('',#14141);
#4109=VERTEX_POINT('',#14145);
#4110=VERTEX_POINT('',#14147);
#4111=VERTEX_POINT('',#14155);
#4112=VERTEX_POINT('',#14157);
#4113=VERTEX_POINT('',#14161);
#4114=VERTEX_POINT('',#14163);
#4115=VERTEX_POINT('',#14167);
#4116=VERTEX_POINT('',#14169);
#4117=VERTEX_POINT('',#14173);
#4118=VERTEX_POINT('',#14175);
#4824=EDGE_CURVE('',#4013,#4013,#3564,.T.);
#4825=EDGE_CURVE('',#4013,#4014,#2116,.T.);
#4826=EDGE_CURVE('',#4014,#4014,#3565,.T.);
#4827=EDGE_CURVE('',#4015,#4015,#3566,.T.);
#4828=EDGE_CURVE('',#4015,#4016,#2117,.T.);
#4829=EDGE_CURVE('',#4016,#4016,#3567,.T.);
#4830=EDGE_CURVE('',#4017,#4017,#3568,.T.);
#4831=EDGE_CURVE('',#4017,#4018,#2118,.T.);
#4832=EDGE_CURVE('',#4018,#4018,#3569,.T.);
#4833=EDGE_CURVE('',#4019,#4019,#3570,.T.);
#4834=EDGE_CURVE('',#4019,#4020,#2119,.T.);
#4835=EDGE_CURVE('',#4020,#4020,#3571,.T.);
#4836=EDGE_CURVE('',#4021,#4021,#3572,.T.);
#4837=EDGE_CURVE('',#4021,#4022,#2120,.T.);
#4838=EDGE_CURVE('',#4022,#4022,#3573,.T.);
#4839=EDGE_CURVE('',#4023,#4023,#3574,.T.);
#4840=EDGE_CURVE('',#4023,#4024,#2121,.T.);
#4841=EDGE_CURVE('',#4024,#4024,#3575,.T.);
#4842=EDGE_CURVE('',#4025,#4025,#3576,.T.);
#4843=EDGE_CURVE('',#4025,#4026,#2122,.T.);
#4844=EDGE_CURVE('',#4026,#4026,#3577,.T.);
#4845=EDGE_CURVE('',#4027,#4027,#3578,.T.);
#4846=EDGE_CURVE('',#4027,#4028,#2123,.T.);
#4847=EDGE_CURVE('',#4028,#4028,#3579,.T.);
#4848=EDGE_CURVE('',#4029,#4029,#3580,.T.);
#4849=EDGE_CURVE('',#4029,#4030,#2124,.T.);
#4850=EDGE_CURVE('',#4030,#4030,#3581,.T.);
#4851=EDGE_CURVE('',#4031,#4031,#3582,.T.);
#4852=EDGE_CURVE('',#4031,#4032,#2125,.T.);
#4853=EDGE_CURVE('',#4032,#4032,#3583,.T.);
#4854=EDGE_CURVE('',#4033,#4033,#3584,.T.);
#4855=EDGE_CURVE('',#4033,#4034,#2126,.T.);
#4856=EDGE_CURVE('',#4034,#4034,#3585,.T.);
#4857=EDGE_CURVE('',#4035,#4036,#2127,.T.);
#4858=EDGE_CURVE('',#4036,#4037,#3586,.T.);
#4859=EDGE_CURVE('',#4038,#4037,#2128,.T.);
#4860=EDGE_CURVE('',#4038,#4035,#2129,.T.);
#4861=EDGE_CURVE('',#4039,#4040,#2130,.T.);
#4862=EDGE_CURVE('',#4039,#4041,#3587,.T.);
#4863=EDGE_CURVE('',#4041,#4042,#2131,.T.);
#4864=EDGE_CURVE('',#4042,#4040,#2132,.T.);
#4865=EDGE_CURVE('',#4043,#4037,#2133,.T.);
#4866=EDGE_CURVE('',#4037,#4039,#2134,.T.);
#4867=EDGE_CURVE('',#4044,#4039,#2135,.T.);
#4868=EDGE_CURVE('',#4044,#4043,#2136,.T.);
#4869=EDGE_CURVE('',#4045,#4046,#2137,.T.);
#4870=EDGE_CURVE('',#4047,#4045,#2138,.T.);
#4871=EDGE_CURVE('',#4048,#4047,#2139,.T.);
#4872=EDGE_CURVE('',#4048,#4046,#2140,.T.);
#4873=EDGE_CURVE('',#4049,#4050,#2141,.T.);
#4874=EDGE_CURVE('',#4050,#4044,#3588,.T.);
#4875=EDGE_CURVE('',#4051,#4044,#2142,.T.);
#4876=EDGE_CURVE('',#4051,#4049,#2143,.T.);
#4877=EDGE_CURVE('',#4052,#4043,#2144,.T.);
#4878=EDGE_CURVE('',#4043,#4053,#3589,.T.);
#4879=EDGE_CURVE('',#4054,#4053,#2145,.T.);
#4880=EDGE_CURVE('',#4054,#4052,#2146,.T.);
#4881=EDGE_CURVE('',#4055,#4056,#2147,.T.);
#4882=EDGE_CURVE('',#4057,#4055,#3590,.T.);
#4883=EDGE_CURVE('',#4058,#4057,#2148,.T.);
#4884=EDGE_CURVE('',#4058,#4056,#3591,.T.);
#4885=EDGE_CURVE('',#4055,#4059,#2149,.T.);
#4886=EDGE_CURVE('',#4056,#4060,#2150,.T.);
#4887=EDGE_CURVE('',#4060,#4059,#2151,.T.);
#4888=EDGE_CURVE('',#4061,#4062,#2152,.T.);
#4889=EDGE_CURVE('',#4061,#4063,#3592,.T.);
#4890=EDGE_CURVE('',#4064,#4063,#2153,.T.);
#4891=EDGE_CURVE('',#4062,#4064,#3593,.T.);
#4892=EDGE_CURVE('',#4065,#4061,#2154,.T.);
#4893=EDGE_CURVE('',#4066,#4062,#2155,.T.);
#4894=EDGE_CURVE('',#4066,#4065,#2156,.T.);
#4895=EDGE_CURVE('',#4067,#4068,#2157,.T.);
#4896=EDGE_CURVE('',#4059,#4067,#3594,.T.);
#4897=EDGE_CURVE('',#4060,#4068,#3595,.T.);
#4898=EDGE_CURVE('',#4067,#4069,#2158,.T.);
#4899=EDGE_CURVE('',#4068,#4070,#2159,.T.);
#4900=EDGE_CURVE('',#4070,#4069,#2160,.T.);
#4901=EDGE_CURVE('',#4071,#4072,#2161,.T.);
#4902=EDGE_CURVE('',#4071,#4073,#3596,.T.);
#4903=EDGE_CURVE('',#4074,#4073,#2162,.T.);
#4904=EDGE_CURVE('',#4072,#4074,#3597,.T.);
#4905=EDGE_CURVE('',#4063,#4071,#2163,.T.);
#4906=EDGE_CURVE('',#4064,#4072,#2164,.T.);
#4907=EDGE_CURVE('',#4069,#4051,#3598,.T.);
#4908=EDGE_CURVE('',#4070,#4049,#3599,.T.);
#4909=EDGE_CURVE('',#4075,#4076,#2165,.T.);
#4910=EDGE_CURVE('',#4075,#4040,#3600,.T.);
#4911=EDGE_CURVE('',#4076,#4042,#3601,.T.);
#4912=EDGE_CURVE('',#4073,#4075,#2166,.T.);
#4913=EDGE_CURVE('',#4074,#4076,#2167,.T.);
#4914=EDGE_CURVE('',#4077,#4078,#2168,.T.);
#4915=EDGE_CURVE('',#4052,#4077,#3602,.T.);
#4916=EDGE_CURVE('',#4054,#4078,#3603,.T.);
#4917=EDGE_CURVE('',#4077,#4079,#2169,.T.);
#4918=EDGE_CURVE('',#4078,#4080,#2170,.T.);
#4919=EDGE_CURVE('',#4080,#4079,#2171,.T.);
#4920=EDGE_CURVE('',#4038,#4081,#3604,.T.);
#4921=EDGE_CURVE('',#4082,#4081,#2172,.T.);
#4922=EDGE_CURVE('',#4035,#4082,#3605,.T.);
#4923=EDGE_CURVE('',#4083,#4084,#2173,.T.);
#4924=EDGE_CURVE('',#4079,#4083,#3606,.T.);
#4925=EDGE_CURVE('',#4080,#4084,#3607,.T.);
#4926=EDGE_CURVE('',#4083,#4085,#2174,.T.);
#4927=EDGE_CURVE('',#4084,#4086,#2175,.T.);
#4928=EDGE_CURVE('',#4085,#4086,#2176,.T.);
#4929=EDGE_CURVE('',#4087,#4088,#2177,.T.);
#4930=EDGE_CURVE('',#4087,#4089,#3608,.T.);
#4931=EDGE_CURVE('',#4090,#4089,#2178,.T.);
#4932=EDGE_CURVE('',#4088,#4090,#3609,.T.);
#4933=EDGE_CURVE('',#4081,#4087,#2179,.T.);
#4934=EDGE_CURVE('',#4082,#4088,#2180,.T.);
#4935=EDGE_CURVE('',#4090,#4091,#2181,.T.);
#4936=EDGE_CURVE('',#4086,#4091,#2182,.T.);
#4937=EDGE_CURVE('',#4084,#4090,#2183,.T.);
#4938=EDGE_CURVE('',#4092,#4091,#2184,.T.);
#4939=EDGE_CURVE('',#4085,#4092,#2185,.T.);
#4940=EDGE_CURVE('',#4089,#4092,#2186,.T.);
#4941=EDGE_CURVE('',#4083,#4089,#2187,.T.);
#4942=EDGE_CURVE('',#4079,#4087,#2188,.T.);
#4943=EDGE_CURVE('',#4077,#4081,#2189,.T.);
#4944=EDGE_CURVE('',#4069,#4075,#2190,.T.);
#4945=EDGE_CURVE('',#4067,#4073,#2191,.T.);
#4946=EDGE_CURVE('',#4059,#4071,#2192,.T.);
#4947=EDGE_CURVE('',#4055,#4063,#2193,.T.);
#4948=EDGE_CURVE('',#4057,#4061,#2194,.T.);
#4949=EDGE_CURVE('',#4093,#4065,#2195,.T.);
#4950=EDGE_CURVE('',#4093,#4057,#2196,.T.);
#4951=EDGE_CURVE('',#4094,#4066,#2197,.T.);
#4952=EDGE_CURVE('',#4094,#4093,#2198,.T.);
#4953=EDGE_CURVE('',#4058,#4062,#2199,.T.);
#4954=EDGE_CURVE('',#4094,#4058,#2200,.T.);
#4955=EDGE_CURVE('',#4056,#4064,#2201,.T.);
#4956=EDGE_CURVE('',#4060,#4072,#2202,.T.);
#4957=EDGE_CURVE('',#4068,#4074,#2203,.T.);
#4958=EDGE_CURVE('',#4070,#4076,#2204,.T.);
#4959=EDGE_CURVE('',#4046,#4041,#2205,.T.);
#4960=EDGE_CURVE('',#4050,#4048,#2206,.T.);
#4961=EDGE_CURVE('',#4078,#4082,#2207,.T.);
#4962=EDGE_CURVE('',#4053,#4047,#2208,.T.);
#4963=EDGE_CURVE('',#4036,#4045,#2209,.T.);
#4964=EDGE_CURVE('',#4080,#4088,#2210,.T.);
#4965=EDGE_CURVE('',#4053,#4095,#3610,.T.);
#4966=EDGE_CURVE('',#4096,#4095,#2211,.T.);
#4967=EDGE_CURVE('',#4047,#4096,#3611,.T.);
#4968=EDGE_CURVE('',#4097,#4050,#3612,.T.);
#4969=EDGE_CURVE('',#4098,#4048,#3613,.T.);
#4970=EDGE_CURVE('',#4098,#4097,#2212,.T.);
#4971=EDGE_CURVE('',#4097,#4095,#2213,.T.);
#4972=EDGE_CURVE('',#4096,#4098,#2214,.T.);
#4973=EDGE_CURVE('',#4098,#4099,#2215,.T.);
#4974=EDGE_CURVE('',#4099,#4100,#2216,.T.);
#4975=EDGE_CURVE('',#4097,#4100,#2217,.T.);
#4976=EDGE_CURVE('',#4101,#4095,#2218,.T.);
#4977=EDGE_CURVE('',#4101,#4102,#2219,.T.);
#4978=EDGE_CURVE('',#4102,#4096,#2220,.T.);
#4979=EDGE_CURVE('',#4100,#4103,#2221,.T.);
#4980=EDGE_CURVE('',#4103,#4104,#2222,.T.);
#4981=EDGE_CURVE('',#4104,#4101,#2223,.T.);
#4982=EDGE_CURVE('',#4105,#4102,#2224,.T.);
#4983=EDGE_CURVE('',#4106,#4105,#2225,.T.);
#4984=EDGE_CURVE('',#4099,#4106,#2226,.T.);
#4985=EDGE_CURVE('',#4105,#4104,#2227,.T.);
#4986=EDGE_CURVE('',#4106,#4103,#2228,.T.);
#4987=EDGE_CURVE('',#4046,#4107,#3614,.T.);
#4988=EDGE_CURVE('',#4041,#4108,#3615,.T.);
#4989=EDGE_CURVE('',#4107,#4108,#2229,.T.);
#4990=EDGE_CURVE('',#4109,#4036,#3616,.T.);
#4991=EDGE_CURVE('',#4110,#4045,#3617,.T.);
#4992=EDGE_CURVE('',#4110,#4109,#2230,.T.);
#4993=EDGE_CURVE('',#4109,#4108,#2231,.T.);
#4994=EDGE_CURVE('',#4107,#4110,#2232,.T.);
#4995=EDGE_CURVE('',#4111,#4108,#2233,.T.);
#4996=EDGE_CURVE('',#4112,#4111,#2234,.T.);
#4997=EDGE_CURVE('',#4112,#4107,#2235,.T.);
#4998=EDGE_CURVE('',#4110,#4113,#2236,.T.);
#4999=EDGE_CURVE('',#4114,#4113,#2237,.T.);
#5000=EDGE_CURVE('',#4109,#4114,#2238,.T.);
#5001=EDGE_CURVE('',#4114,#4115,#2239,.T.);
#5002=EDGE_CURVE('',#4115,#4116,#2240,.T.);
#5003=EDGE_CURVE('',#4116,#4111,#2241,.T.);
#5004=EDGE_CURVE('',#4117,#4112,#2242,.T.);
#5005=EDGE_CURVE('',#4118,#4117,#2243,.T.);
#5006=EDGE_CURVE('',#4113,#4118,#2244,.T.);
#5007=EDGE_CURVE('',#4118,#4115,#2245,.T.);
#5008=EDGE_CURVE('',#4117,#4116,#2246,.T.);
#6152=ORIENTED_EDGE('',*,*,#4824,.T.);
#6153=ORIENTED_EDGE('',*,*,#4825,.T.);
#6154=ORIENTED_EDGE('',*,*,#4826,.T.);
#6155=ORIENTED_EDGE('',*,*,#4825,.F.);
#6156=ORIENTED_EDGE('',*,*,#4827,.T.);
#6157=ORIENTED_EDGE('',*,*,#4828,.T.);
#6158=ORIENTED_EDGE('',*,*,#4829,.T.);
#6159=ORIENTED_EDGE('',*,*,#4828,.F.);
#6160=ORIENTED_EDGE('',*,*,#4830,.F.);
#6161=ORIENTED_EDGE('',*,*,#4831,.T.);
#6162=ORIENTED_EDGE('',*,*,#4832,.T.);
#6163=ORIENTED_EDGE('',*,*,#4831,.F.);
#6164=ORIENTED_EDGE('',*,*,#4833,.F.);
#6165=ORIENTED_EDGE('',*,*,#4834,.T.);
#6166=ORIENTED_EDGE('',*,*,#4835,.T.);
#6167=ORIENTED_EDGE('',*,*,#4834,.F.);
#6168=ORIENTED_EDGE('',*,*,#4836,.F.);
#6169=ORIENTED_EDGE('',*,*,#4837,.T.);
#6170=ORIENTED_EDGE('',*,*,#4838,.T.);
#6171=ORIENTED_EDGE('',*,*,#4837,.F.);
#6172=ORIENTED_EDGE('',*,*,#4839,.F.);
#6173=ORIENTED_EDGE('',*,*,#4840,.T.);
#6174=ORIENTED_EDGE('',*,*,#4841,.T.);
#6175=ORIENTED_EDGE('',*,*,#4840,.F.);
#6176=ORIENTED_EDGE('',*,*,#4842,.F.);
#6177=ORIENTED_EDGE('',*,*,#4843,.T.);
#6178=ORIENTED_EDGE('',*,*,#4844,.T.);
#6179=ORIENTED_EDGE('',*,*,#4843,.F.);
#6180=ORIENTED_EDGE('',*,*,#4845,.F.);
#6181=ORIENTED_EDGE('',*,*,#4846,.T.);
#6182=ORIENTED_EDGE('',*,*,#4847,.T.);
#6183=ORIENTED_EDGE('',*,*,#4846,.F.);
#6184=ORIENTED_EDGE('',*,*,#4848,.F.);
#6185=ORIENTED_EDGE('',*,*,#4849,.T.);
#6186=ORIENTED_EDGE('',*,*,#4850,.T.);
#6187=ORIENTED_EDGE('',*,*,#4849,.F.);
#6188=ORIENTED_EDGE('',*,*,#4851,.F.);
#6189=ORIENTED_EDGE('',*,*,#4852,.T.);
#6190=ORIENTED_EDGE('',*,*,#4853,.T.);
#6191=ORIENTED_EDGE('',*,*,#4852,.F.);
#6192=ORIENTED_EDGE('',*,*,#4854,.F.);
#6193=ORIENTED_EDGE('',*,*,#4855,.T.);
#6194=ORIENTED_EDGE('',*,*,#4856,.T.);
#6195=ORIENTED_EDGE('',*,*,#4855,.F.);
#6196=ORIENTED_EDGE('',*,*,#4857,.T.);
#6197=ORIENTED_EDGE('',*,*,#4858,.T.);
#6198=ORIENTED_EDGE('',*,*,#4859,.F.);
#6199=ORIENTED_EDGE('',*,*,#4860,.T.);
#6200=ORIENTED_EDGE('',*,*,#4861,.F.);
#6201=ORIENTED_EDGE('',*,*,#4862,.T.);
#6202=ORIENTED_EDGE('',*,*,#4863,.T.);
#6203=ORIENTED_EDGE('',*,*,#4864,.T.);
#6204=ORIENTED_EDGE('',*,*,#4865,.T.);
#6205=ORIENTED_EDGE('',*,*,#4866,.T.);
#6206=ORIENTED_EDGE('',*,*,#4867,.F.);
#6207=ORIENTED_EDGE('',*,*,#4868,.T.);
#6208=ORIENTED_EDGE('',*,*,#4869,.F.);
#6209=ORIENTED_EDGE('',*,*,#4870,.F.);
#6210=ORIENTED_EDGE('',*,*,#4871,.F.);
#6211=ORIENTED_EDGE('',*,*,#4872,.T.);
#6212=ORIENTED_EDGE('',*,*,#4873,.T.);
#6213=ORIENTED_EDGE('',*,*,#4874,.T.);
#6214=ORIENTED_EDGE('',*,*,#4875,.F.);
#6215=ORIENTED_EDGE('',*,*,#4876,.T.);
#6216=ORIENTED_EDGE('',*,*,#4877,.T.);
#6217=ORIENTED_EDGE('',*,*,#4878,.T.);
#6218=ORIENTED_EDGE('',*,*,#4879,.F.);
#6219=ORIENTED_EDGE('',*,*,#4880,.T.);
#6220=ORIENTED_EDGE('',*,*,#4881,.F.);
#6221=ORIENTED_EDGE('',*,*,#4882,.F.);
#6222=ORIENTED_EDGE('',*,*,#4883,.F.);
#6223=ORIENTED_EDGE('',*,*,#4884,.T.);
#6224=ORIENTED_EDGE('',*,*,#4885,.F.);
#6225=ORIENTED_EDGE('',*,*,#4881,.T.);
#6226=ORIENTED_EDGE('',*,*,#4886,.T.);
#6227=ORIENTED_EDGE('',*,*,#4887,.T.);
#6228=ORIENTED_EDGE('',*,*,#4888,.F.);
#6229=ORIENTED_EDGE('',*,*,#4889,.T.);
#6230=ORIENTED_EDGE('',*,*,#4890,.F.);
#6231=ORIENTED_EDGE('',*,*,#4891,.F.);
#6232=ORIENTED_EDGE('',*,*,#4892,.T.);
#6233=ORIENTED_EDGE('',*,*,#4888,.T.);
#6234=ORIENTED_EDGE('',*,*,#4893,.F.);
#6235=ORIENTED_EDGE('',*,*,#4894,.T.);
#6236=ORIENTED_EDGE('',*,*,#4895,.F.);
#6237=ORIENTED_EDGE('',*,*,#4896,.F.);
#6238=ORIENTED_EDGE('',*,*,#4887,.F.);
#6239=ORIENTED_EDGE('',*,*,#4897,.T.);
#6240=ORIENTED_EDGE('',*,*,#4898,.F.);
#6241=ORIENTED_EDGE('',*,*,#4895,.T.);
#6242=ORIENTED_EDGE('',*,*,#4899,.T.);
#6243=ORIENTED_EDGE('',*,*,#4900,.T.);
#6244=ORIENTED_EDGE('',*,*,#4901,.F.);
#6245=ORIENTED_EDGE('',*,*,#4902,.T.);
#6246=ORIENTED_EDGE('',*,*,#4903,.F.);
#6247=ORIENTED_EDGE('',*,*,#4904,.F.);
#6248=ORIENTED_EDGE('',*,*,#4905,.T.);
#6249=ORIENTED_EDGE('',*,*,#4901,.T.);
#6250=ORIENTED_EDGE('',*,*,#4906,.F.);
#6251=ORIENTED_EDGE('',*,*,#4890,.T.);
#6252=ORIENTED_EDGE('',*,*,#4876,.F.);
#6253=ORIENTED_EDGE('',*,*,#4907,.F.);
#6254=ORIENTED_EDGE('',*,*,#4900,.F.);
#6255=ORIENTED_EDGE('',*,*,#4908,.T.);
#6256=ORIENTED_EDGE('',*,*,#4909,.F.);
#6257=ORIENTED_EDGE('',*,*,#4910,.T.);
#6258=ORIENTED_EDGE('',*,*,#4864,.F.);
#6259=ORIENTED_EDGE('',*,*,#4911,.F.);
#6260=ORIENTED_EDGE('',*,*,#4912,.T.);
#6261=ORIENTED_EDGE('',*,*,#4909,.T.);
#6262=ORIENTED_EDGE('',*,*,#4913,.F.);
#6263=ORIENTED_EDGE('',*,*,#4903,.T.);
#6264=ORIENTED_EDGE('',*,*,#4914,.F.);
#6265=ORIENTED_EDGE('',*,*,#4915,.F.);
#6266=ORIENTED_EDGE('',*,*,#4880,.F.);
#6267=ORIENTED_EDGE('',*,*,#4916,.T.);
#6268=ORIENTED_EDGE('',*,*,#4917,.F.);
#6269=ORIENTED_EDGE('',*,*,#4914,.T.);
#6270=ORIENTED_EDGE('',*,*,#4918,.T.);
#6271=ORIENTED_EDGE('',*,*,#4919,.T.);
#6272=ORIENTED_EDGE('',*,*,#4860,.F.);
#6273=ORIENTED_EDGE('',*,*,#4920,.T.);
#6274=ORIENTED_EDGE('',*,*,#4921,.F.);
#6275=ORIENTED_EDGE('',*,*,#4922,.F.);
#6276=ORIENTED_EDGE('',*,*,#4923,.F.);
#6277=ORIENTED_EDGE('',*,*,#4924,.F.);
#6278=ORIENTED_EDGE('',*,*,#4919,.F.);
#6279=ORIENTED_EDGE('',*,*,#4925,.T.);
#6280=ORIENTED_EDGE('',*,*,#4926,.F.);
#6281=ORIENTED_EDGE('',*,*,#4923,.T.);
#6282=ORIENTED_EDGE('',*,*,#4927,.T.);
#6283=ORIENTED_EDGE('',*,*,#4928,.F.);
#6284=ORIENTED_EDGE('',*,*,#4929,.F.);
#6285=ORIENTED_EDGE('',*,*,#4930,.T.);
#6286=ORIENTED_EDGE('',*,*,#4931,.F.);
#6287=ORIENTED_EDGE('',*,*,#4932,.F.);
#6288=ORIENTED_EDGE('',*,*,#4933,.T.);
#6289=ORIENTED_EDGE('',*,*,#4929,.T.);
#6290=ORIENTED_EDGE('',*,*,#4934,.F.);
#6291=ORIENTED_EDGE('',*,*,#4921,.T.);
#6292=ORIENTED_EDGE('',*,*,#4935,.T.);
#6293=ORIENTED_EDGE('',*,*,#4936,.F.);
#6294=ORIENTED_EDGE('',*,*,#4927,.F.);
#6295=ORIENTED_EDGE('',*,*,#4937,.T.);
#6296=ORIENTED_EDGE('',*,*,#4836,.T.);
#6297=ORIENTED_EDGE('',*,*,#4839,.T.);
#6298=ORIENTED_EDGE('',*,*,#4845,.T.);
#6299=ORIENTED_EDGE('',*,*,#4848,.T.);
#6300=ORIENTED_EDGE('',*,*,#4938,.F.);
#6301=ORIENTED_EDGE('',*,*,#4939,.F.);
#6302=ORIENTED_EDGE('',*,*,#4928,.T.);
#6303=ORIENTED_EDGE('',*,*,#4936,.T.);
#6304=ORIENTED_EDGE('',*,*,#4940,.F.);
#6305=ORIENTED_EDGE('',*,*,#4941,.F.);
#6306=ORIENTED_EDGE('',*,*,#4926,.T.);
#6307=ORIENTED_EDGE('',*,*,#4939,.T.);
#6308=ORIENTED_EDGE('',*,*,#4838,.F.);
#6309=ORIENTED_EDGE('',*,*,#4841,.F.);
#6310=ORIENTED_EDGE('',*,*,#4847,.F.);
#6311=ORIENTED_EDGE('',*,*,#4850,.F.);
#6312=ORIENTED_EDGE('',*,*,#4930,.F.);
#6313=ORIENTED_EDGE('',*,*,#4942,.F.);
#6314=ORIENTED_EDGE('',*,*,#4924,.T.);
#6315=ORIENTED_EDGE('',*,*,#4941,.T.);
#6316=ORIENTED_EDGE('',*,*,#4933,.F.);
#6317=ORIENTED_EDGE('',*,*,#4943,.F.);
#6318=ORIENTED_EDGE('',*,*,#4917,.T.);
#6319=ORIENTED_EDGE('',*,*,#4942,.T.);
#6320=ORIENTED_EDGE('',*,*,#4920,.F.);
#6321=ORIENTED_EDGE('',*,*,#4859,.T.);
#6322=ORIENTED_EDGE('',*,*,#4865,.F.);
#6323=ORIENTED_EDGE('',*,*,#4877,.F.);
#6324=ORIENTED_EDGE('',*,*,#4915,.T.);
#6325=ORIENTED_EDGE('',*,*,#4943,.T.);
#6326=ORIENTED_EDGE('',*,*,#4910,.F.);
#6327=ORIENTED_EDGE('',*,*,#4944,.F.);
#6328=ORIENTED_EDGE('',*,*,#4907,.T.);
#6329=ORIENTED_EDGE('',*,*,#4875,.T.);
#6330=ORIENTED_EDGE('',*,*,#4867,.T.);
#6331=ORIENTED_EDGE('',*,*,#4861,.T.);
#6332=ORIENTED_EDGE('',*,*,#4912,.F.);
#6333=ORIENTED_EDGE('',*,*,#4945,.F.);
#6334=ORIENTED_EDGE('',*,*,#4898,.T.);
#6335=ORIENTED_EDGE('',*,*,#4944,.T.);
#6336=ORIENTED_EDGE('',*,*,#4902,.F.);
#6337=ORIENTED_EDGE('',*,*,#4946,.F.);
#6338=ORIENTED_EDGE('',*,*,#4896,.T.);
#6339=ORIENTED_EDGE('',*,*,#4945,.T.);
#6340=ORIENTED_EDGE('',*,*,#4905,.F.);
#6341=ORIENTED_EDGE('',*,*,#4947,.F.);
#6342=ORIENTED_EDGE('',*,*,#4885,.T.);
#6343=ORIENTED_EDGE('',*,*,#4946,.T.);
#6344=ORIENTED_EDGE('',*,*,#4889,.F.);
#6345=ORIENTED_EDGE('',*,*,#4948,.F.);
#6346=ORIENTED_EDGE('',*,*,#4882,.T.);
#6347=ORIENTED_EDGE('',*,*,#4947,.T.);
#6348=ORIENTED_EDGE('',*,*,#4892,.F.);
#6349=ORIENTED_EDGE('',*,*,#4949,.F.);
#6350=ORIENTED_EDGE('',*,*,#4950,.T.);
#6351=ORIENTED_EDGE('',*,*,#4948,.T.);
#6352=ORIENTED_EDGE('',*,*,#4844,.F.);
#6353=ORIENTED_EDGE('',*,*,#4853,.F.);
#6354=ORIENTED_EDGE('',*,*,#4856,.F.);
#6355=ORIENTED_EDGE('',*,*,#4894,.F.);
#6356=ORIENTED_EDGE('',*,*,#4951,.F.);
#6357=ORIENTED_EDGE('',*,*,#4952,.T.);
#6358=ORIENTED_EDGE('',*,*,#4949,.T.);
#6359=ORIENTED_EDGE('',*,*,#4893,.T.);
#6360=ORIENTED_EDGE('',*,*,#4953,.F.);
#6361=ORIENTED_EDGE('',*,*,#4954,.F.);
#6362=ORIENTED_EDGE('',*,*,#4951,.T.);
#6363=ORIENTED_EDGE('',*,*,#4842,.T.);
#6364=ORIENTED_EDGE('',*,*,#4851,.T.);
#6365=ORIENTED_EDGE('',*,*,#4854,.T.);
#6366=ORIENTED_EDGE('',*,*,#4891,.T.);
#6367=ORIENTED_EDGE('',*,*,#4955,.F.);
#6368=ORIENTED_EDGE('',*,*,#4884,.F.);
#6369=ORIENTED_EDGE('',*,*,#4953,.T.);
#6370=ORIENTED_EDGE('',*,*,#4906,.T.);
#6371=ORIENTED_EDGE('',*,*,#4956,.F.);
#6372=ORIENTED_EDGE('',*,*,#4886,.F.);
#6373=ORIENTED_EDGE('',*,*,#4955,.T.);
#6374=ORIENTED_EDGE('',*,*,#4904,.T.);
#6375=ORIENTED_EDGE('',*,*,#4957,.F.);
#6376=ORIENTED_EDGE('',*,*,#4897,.F.);
#6377=ORIENTED_EDGE('',*,*,#4956,.T.);
#6378=ORIENTED_EDGE('',*,*,#4913,.T.);
#6379=ORIENTED_EDGE('',*,*,#4958,.F.);
#6380=ORIENTED_EDGE('',*,*,#4899,.F.);
#6381=ORIENTED_EDGE('',*,*,#4957,.T.);
#6382=ORIENTED_EDGE('',*,*,#4911,.T.);
#6383=ORIENTED_EDGE('',*,*,#4863,.F.);
#6384=ORIENTED_EDGE('',*,*,#4959,.F.);
#6385=ORIENTED_EDGE('',*,*,#4872,.F.);
#6386=ORIENTED_EDGE('',*,*,#4960,.F.);
#6387=ORIENTED_EDGE('',*,*,#4873,.F.);
#6388=ORIENTED_EDGE('',*,*,#4908,.F.);
#6389=ORIENTED_EDGE('',*,*,#4958,.T.);
#6390=ORIENTED_EDGE('',*,*,#4922,.T.);
#6391=ORIENTED_EDGE('',*,*,#4961,.F.);
#6392=ORIENTED_EDGE('',*,*,#4916,.F.);
#6393=ORIENTED_EDGE('',*,*,#4879,.T.);
#6394=ORIENTED_EDGE('',*,*,#4962,.T.);
#6395=ORIENTED_EDGE('',*,*,#4870,.T.);
#6396=ORIENTED_EDGE('',*,*,#4963,.F.);
#6397=ORIENTED_EDGE('',*,*,#4857,.F.);
#6398=ORIENTED_EDGE('',*,*,#4934,.T.);
#6399=ORIENTED_EDGE('',*,*,#4964,.F.);
#6400=ORIENTED_EDGE('',*,*,#4918,.F.);
#6401=ORIENTED_EDGE('',*,*,#4961,.T.);
#6402=ORIENTED_EDGE('',*,*,#4932,.T.);
#6403=ORIENTED_EDGE('',*,*,#4937,.F.);
#6404=ORIENTED_EDGE('',*,*,#4925,.F.);
#6405=ORIENTED_EDGE('',*,*,#4964,.T.);
#6406=ORIENTED_EDGE('',*,*,#4954,.T.);
#6407=ORIENTED_EDGE('',*,*,#4883,.T.);
#6408=ORIENTED_EDGE('',*,*,#4950,.F.);
#6409=ORIENTED_EDGE('',*,*,#4952,.F.);
#6410=ORIENTED_EDGE('',*,*,#4935,.F.);
#6411=ORIENTED_EDGE('',*,*,#4931,.T.);
#6412=ORIENTED_EDGE('',*,*,#4940,.T.);
#6413=ORIENTED_EDGE('',*,*,#4938,.T.);
#6414=ORIENTED_EDGE('',*,*,#4962,.F.);
#6415=ORIENTED_EDGE('',*,*,#4965,.T.);
#6416=ORIENTED_EDGE('',*,*,#4966,.F.);
#6417=ORIENTED_EDGE('',*,*,#4967,.F.);
#6418=ORIENTED_EDGE('',*,*,#4968,.T.);
#6419=ORIENTED_EDGE('',*,*,#4960,.T.);
#6420=ORIENTED_EDGE('',*,*,#4969,.F.);
#6421=ORIENTED_EDGE('',*,*,#4970,.T.);
#6422=ORIENTED_EDGE('',*,*,#4868,.F.);
#6423=ORIENTED_EDGE('',*,*,#4874,.F.);
#6424=ORIENTED_EDGE('',*,*,#4968,.F.);
#6425=ORIENTED_EDGE('',*,*,#4971,.T.);
#6426=ORIENTED_EDGE('',*,*,#4965,.F.);
#6427=ORIENTED_EDGE('',*,*,#4878,.F.);
#6428=ORIENTED_EDGE('',*,*,#4871,.T.);
#6429=ORIENTED_EDGE('',*,*,#4967,.T.);
#6430=ORIENTED_EDGE('',*,*,#4972,.T.);
#6431=ORIENTED_EDGE('',*,*,#4969,.T.);
#6432=ORIENTED_EDGE('',*,*,#4973,.T.);
#6433=ORIENTED_EDGE('',*,*,#4974,.T.);
#6434=ORIENTED_EDGE('',*,*,#4975,.F.);
#6435=ORIENTED_EDGE('',*,*,#4970,.F.);
#6436=ORIENTED_EDGE('',*,*,#4966,.T.);
#6437=ORIENTED_EDGE('',*,*,#4976,.F.);
#6438=ORIENTED_EDGE('',*,*,#4977,.T.);
#6439=ORIENTED_EDGE('',*,*,#4978,.T.);
#6440=ORIENTED_EDGE('',*,*,#4971,.F.);
#6441=ORIENTED_EDGE('',*,*,#4975,.T.);
#6442=ORIENTED_EDGE('',*,*,#4979,.T.);
#6443=ORIENTED_EDGE('',*,*,#4980,.T.);
#6444=ORIENTED_EDGE('',*,*,#4981,.T.);
#6445=ORIENTED_EDGE('',*,*,#4976,.T.);
#6446=ORIENTED_EDGE('',*,*,#4826,.F.);
#6447=ORIENTED_EDGE('',*,*,#4829,.F.);
#6448=ORIENTED_EDGE('',*,*,#4973,.F.);
#6449=ORIENTED_EDGE('',*,*,#4972,.F.);
#6450=ORIENTED_EDGE('',*,*,#4978,.F.);
#6451=ORIENTED_EDGE('',*,*,#4982,.F.);
#6452=ORIENTED_EDGE('',*,*,#4983,.F.);
#6453=ORIENTED_EDGE('',*,*,#4984,.F.);
#6454=ORIENTED_EDGE('',*,*,#4824,.F.);
#6455=ORIENTED_EDGE('',*,*,#4827,.F.);
#6456=ORIENTED_EDGE('',*,*,#4982,.T.);
#6457=ORIENTED_EDGE('',*,*,#4977,.F.);
#6458=ORIENTED_EDGE('',*,*,#4981,.F.);
#6459=ORIENTED_EDGE('',*,*,#4985,.F.);
#6460=ORIENTED_EDGE('',*,*,#4980,.F.);
#6461=ORIENTED_EDGE('',*,*,#4986,.F.);
#6462=ORIENTED_EDGE('',*,*,#4983,.T.);
#6463=ORIENTED_EDGE('',*,*,#4985,.T.);
#6464=ORIENTED_EDGE('',*,*,#4979,.F.);
#6465=ORIENTED_EDGE('',*,*,#4974,.F.);
#6466=ORIENTED_EDGE('',*,*,#4984,.T.);
#6467=ORIENTED_EDGE('',*,*,#4986,.T.);
#6468=ORIENTED_EDGE('',*,*,#4987,.F.);
#6469=ORIENTED_EDGE('',*,*,#4959,.T.);
#6470=ORIENTED_EDGE('',*,*,#4988,.T.);
#6471=ORIENTED_EDGE('',*,*,#4989,.F.);
#6472=ORIENTED_EDGE('',*,*,#4990,.T.);
#6473=ORIENTED_EDGE('',*,*,#4963,.T.);
#6474=ORIENTED_EDGE('',*,*,#4991,.F.);
#6475=ORIENTED_EDGE('',*,*,#4992,.T.);
#6476=ORIENTED_EDGE('',*,*,#4866,.F.);
#6477=ORIENTED_EDGE('',*,*,#4858,.F.);
#6478=ORIENTED_EDGE('',*,*,#4990,.F.);
#6479=ORIENTED_EDGE('',*,*,#4993,.T.);
#6480=ORIENTED_EDGE('',*,*,#4988,.F.);
#6481=ORIENTED_EDGE('',*,*,#4862,.F.);
#6482=ORIENTED_EDGE('',*,*,#4869,.T.);
#6483=ORIENTED_EDGE('',*,*,#4987,.T.);
#6484=ORIENTED_EDGE('',*,*,#4994,.T.);
#6485=ORIENTED_EDGE('',*,*,#4991,.T.);
#6486=ORIENTED_EDGE('',*,*,#4995,.F.);
#6487=ORIENTED_EDGE('',*,*,#4996,.F.);
#6488=ORIENTED_EDGE('',*,*,#4997,.T.);
#6489=ORIENTED_EDGE('',*,*,#4989,.T.);
#6490=ORIENTED_EDGE('',*,*,#4992,.F.);
#6491=ORIENTED_EDGE('',*,*,#4998,.T.);
#6492=ORIENTED_EDGE('',*,*,#4999,.F.);
#6493=ORIENTED_EDGE('',*,*,#5000,.F.);
#6494=ORIENTED_EDGE('',*,*,#4993,.F.);
#6495=ORIENTED_EDGE('',*,*,#5000,.T.);
#6496=ORIENTED_EDGE('',*,*,#5001,.T.);
#6497=ORIENTED_EDGE('',*,*,#5002,.T.);
#6498=ORIENTED_EDGE('',*,*,#5003,.T.);
#6499=ORIENTED_EDGE('',*,*,#4995,.T.);
#6500=ORIENTED_EDGE('',*,*,#4830,.T.);
#6501=ORIENTED_EDGE('',*,*,#4833,.T.);
#6502=ORIENTED_EDGE('',*,*,#4998,.F.);
#6503=ORIENTED_EDGE('',*,*,#4994,.F.);
#6504=ORIENTED_EDGE('',*,*,#4997,.F.);
#6505=ORIENTED_EDGE('',*,*,#5004,.F.);
#6506=ORIENTED_EDGE('',*,*,#5005,.F.);
#6507=ORIENTED_EDGE('',*,*,#5006,.F.);
#6508=ORIENTED_EDGE('',*,*,#4832,.F.);
#6509=ORIENTED_EDGE('',*,*,#4835,.F.);
#6510=ORIENTED_EDGE('',*,*,#5006,.T.);
#6511=ORIENTED_EDGE('',*,*,#5007,.T.);
#6512=ORIENTED_EDGE('',*,*,#5001,.F.);
#6513=ORIENTED_EDGE('',*,*,#4999,.T.);
#6514=ORIENTED_EDGE('',*,*,#5003,.F.);
#6515=ORIENTED_EDGE('',*,*,#5008,.F.);
#6516=ORIENTED_EDGE('',*,*,#5004,.T.);
#6517=ORIENTED_EDGE('',*,*,#4996,.T.);
#6518=ORIENTED_EDGE('',*,*,#5002,.F.);
#6519=ORIENTED_EDGE('',*,*,#5007,.F.);
#6520=ORIENTED_EDGE('',*,*,#5005,.T.);
#6521=ORIENTED_EDGE('',*,*,#5008,.T.);
#8808=CYLINDRICAL_SURFACE('',#9751,6.00000000000002);
#8809=CYLINDRICAL_SURFACE('',#9754,6.00000000000001);
#8810=CYLINDRICAL_SURFACE('',#9757,6.00000000000002);
#8811=CYLINDRICAL_SURFACE('',#9760,6.00000000000001);
#8812=CYLINDRICAL_SURFACE('',#9763,6.34999999999999);
#8813=CYLINDRICAL_SURFACE('',#9766,6.35000000000122);
#8814=CYLINDRICAL_SURFACE('',#9769,6.35000000000122);
#8815=CYLINDRICAL_SURFACE('',#9772,6.46290152238551);
#8816=CYLINDRICAL_SURFACE('',#9775,6.4629015223855);
#8817=CYLINDRICAL_SURFACE('',#9778,6.34999999999994);
#8818=CYLINDRICAL_SURFACE('',#9781,6.34999999999994);
#8819=CYLINDRICAL_SURFACE('',#9835,4.);
#8820=CYLINDRICAL_SURFACE('',#9837,4.);
#8821=CYLINDRICAL_SURFACE('',#9838,4.);
#8822=CYLINDRICAL_SURFACE('',#9840,4.);
#8823=CYLINDRICAL_SURFACE('',#9842,4.);
#8824=CYLINDRICAL_SURFACE('',#9846,1.);
#8825=CYLINDRICAL_SURFACE('',#9848,1.);
#8826=CYLINDRICAL_SURFACE('',#9850,1.);
#8827=CYLINDRICAL_SURFACE('',#9851,1.);
#8828=CYLINDRICAL_SURFACE('',#9853,1.);
#8829=CYLINDRICAL_SURFACE('',#9862,4.);
#8830=CYLINDRICAL_SURFACE('',#9863,1.);
#8831=CYLINDRICAL_SURFACE('',#9877,4.);
#8832=CYLINDRICAL_SURFACE('',#9878,1.);
#8980=ADVANCED_FACE('',(#841),#8808,.F.);
#8981=ADVANCED_FACE('',(#842),#8809,.F.);
#8982=ADVANCED_FACE('',(#843),#8810,.F.);
#8983=ADVANCED_FACE('',(#844),#8811,.F.);
#8984=ADVANCED_FACE('',(#845),#8812,.F.);
#8985=ADVANCED_FACE('',(#846),#8813,.F.);
#8986=ADVANCED_FACE('',(#847),#8814,.F.);
#8987=ADVANCED_FACE('',(#848),#8815,.F.);
#8988=ADVANCED_FACE('',(#849),#8816,.F.);
#8989=ADVANCED_FACE('',(#850),#8817,.F.);
#8990=ADVANCED_FACE('',(#851),#8818,.F.);
#8991=ADVANCED_FACE('',(#852),#502,.T.);
#8992=ADVANCED_FACE('',(#853),#503,.T.);
#8993=ADVANCED_FACE('',(#854),#504,.T.);
#8994=ADVANCED_FACE('',(#855),#505,.F.);
#8995=ADVANCED_FACE('',(#856),#506,.T.);
#8996=ADVANCED_FACE('',(#857),#507,.T.);
#8997=ADVANCED_FACE('',(#858),#508,.T.);
#8998=ADVANCED_FACE('',(#859),#509,.T.);
#8999=ADVANCED_FACE('',(#860),#510,.T.);
#9000=ADVANCED_FACE('',(#861),#511,.T.);
#9001=ADVANCED_FACE('',(#862),#512,.T.);
#9002=ADVANCED_FACE('',(#863),#513,.T.);
#9003=ADVANCED_FACE('',(#864),#514,.T.);
#9004=ADVANCED_FACE('',(#865),#515,.T.);
#9005=ADVANCED_FACE('',(#866),#516,.T.);
#9006=ADVANCED_FACE('',(#867),#517,.T.);
#9007=ADVANCED_FACE('',(#868),#518,.T.);
#9008=ADVANCED_FACE('',(#869),#519,.T.);
#9009=ADVANCED_FACE('',(#870),#520,.T.);
#9010=ADVANCED_FACE('',(#871),#521,.T.);
#9011=ADVANCED_FACE('',(#872),#522,.T.);
#9012=ADVANCED_FACE('',(#873),#523,.T.);
#9013=ADVANCED_FACE('',(#874),#524,.T.);
#9014=ADVANCED_FACE('',(#875),#525,.T.);
#9015=ADVANCED_FACE('',(#876,#379,#380,#381,#382),#526,.F.);
#9016=ADVANCED_FACE('',(#877),#527,.T.);
#9017=ADVANCED_FACE('',(#878,#383,#384,#385,#386),#528,.T.);
#9018=ADVANCED_FACE('',(#879),#8819,.T.);
#9019=ADVANCED_FACE('',(#880),#529,.T.);
#9020=ADVANCED_FACE('',(#881),#8820,.T.);
#9021=ADVANCED_FACE('',(#882),#8821,.T.);
#9022=ADVANCED_FACE('',(#883),#530,.T.);
#9023=ADVANCED_FACE('',(#884),#8822,.T.);
#9024=ADVANCED_FACE('',(#885),#531,.T.);
#9025=ADVANCED_FACE('',(#886),#8823,.T.);
#9026=ADVANCED_FACE('',(#887,#387,#388,#389),#532,.T.);
#9027=ADVANCED_FACE('',(#888),#533,.T.);
#9028=ADVANCED_FACE('',(#889,#390,#391,#392),#534,.F.);
#9029=ADVANCED_FACE('',(#890),#8824,.F.);
#9030=ADVANCED_FACE('',(#891),#535,.F.);
#9031=ADVANCED_FACE('',(#892),#8825,.F.);
#9032=ADVANCED_FACE('',(#893),#536,.F.);
#9033=ADVANCED_FACE('',(#894),#8826,.F.);
#9034=ADVANCED_FACE('',(#895),#8827,.F.);
#9035=ADVANCED_FACE('',(#896),#537,.F.);
#9036=ADVANCED_FACE('',(#897),#8828,.F.);
#9037=ADVANCED_FACE('',(#898),#538,.T.);
#9038=ADVANCED_FACE('',(#899),#539,.F.);
#9039=ADVANCED_FACE('',(#900),#540,.T.);
#9040=ADVANCED_FACE('',(#901),#541,.F.);
#9041=ADVANCED_FACE('',(#902),#8829,.T.);
#9042=ADVANCED_FACE('',(#903),#8830,.F.);
#9043=ADVANCED_FACE('',(#904),#542,.F.);
#9044=ADVANCED_FACE('',(#905),#543,.F.);
#9045=ADVANCED_FACE('',(#906,#393,#394),#544,.F.);
#9046=ADVANCED_FACE('',(#907,#395,#396),#545,.T.);
#9047=ADVANCED_FACE('',(#908),#546,.F.);
#9048=ADVANCED_FACE('',(#909),#547,.T.);
#9049=ADVANCED_FACE('',(#910),#548,.T.);
#9050=ADVANCED_FACE('',(#911),#549,.T.);
#9051=ADVANCED_FACE('',(#912),#550,.F.);
#9052=ADVANCED_FACE('',(#913),#8831,.T.);
#9053=ADVANCED_FACE('',(#914),#8832,.F.);
#9054=ADVANCED_FACE('',(#915),#551,.F.);
#9055=ADVANCED_FACE('',(#916),#552,.F.);
#9056=ADVANCED_FACE('',(#917,#397,#398),#553,.F.);
#9057=ADVANCED_FACE('',(#918,#399,#400),#554,.T.);
#9058=ADVANCED_FACE('',(#919),#555,.F.);
#9059=ADVANCED_FACE('',(#920),#556,.T.);
#9060=ADVANCED_FACE('',(#921),#557,.T.);
#9556=CLOSED_SHELL('',(#8980,#8981,#8982,#8983,#8984,#8985,#8986,#8987,
#8988,#8989,#8990,#8991,#8992,#8993,#8994,#8995,#8996,#8997,#8998,#8999,
#9000,#9001,#9002,#9003,#9004,#9005,#9006,#9007,#9008,#9009,#9010,#9011,
#9012,#9013,#9014,#9015,#9016,#9017,#9018,#9019,#9020,#9021,#9022,#9023,
#9024,#9025,#9026,#9027,#9028,#9029,#9030,#9031,#9032,#9033,#9034,#9035,
#9036,#9037,#9038,#9039,#9040,#9041,#9042,#9043,#9044,#9045,#9046,#9047,
#9048,#9049,#9050,#9051,#9052,#9053,#9054,#9055,#9056,#9057,#9058,#9059,
#9060));
#9750=AXIS2_PLACEMENT_3D('',#13810,#10863,#10864);
#9751=AXIS2_PLACEMENT_3D('',#13811,#10865,#10866);
#9752=AXIS2_PLACEMENT_3D('',#13813,#10867,#10868);
#9753=AXIS2_PLACEMENT_3D('',#13816,#10870,#10871);
#9754=AXIS2_PLACEMENT_3D('',#13817,#10872,#10873);
#9755=AXIS2_PLACEMENT_3D('',#13819,#10874,#10875);
#9756=AXIS2_PLACEMENT_3D('',#13822,#10877,#10878);
#9757=AXIS2_PLACEMENT_3D('',#13823,#10879,#10880);
#9758=AXIS2_PLACEMENT_3D('',#13825,#10881,#10882);
#9759=AXIS2_PLACEMENT_3D('',#13828,#10884,#10885);
#9760=AXIS2_PLACEMENT_3D('',#13829,#10886,#10887);
#9761=AXIS2_PLACEMENT_3D('',#13831,#10888,#10889);
#9762=AXIS2_PLACEMENT_3D('',#13834,#10891,#10892);
#9763=AXIS2_PLACEMENT_3D('',#13835,#10893,#10894);
#9764=AXIS2_PLACEMENT_3D('',#13837,#10895,#10896);
#9765=AXIS2_PLACEMENT_3D('',#13840,#10898,#10899);
#9766=AXIS2_PLACEMENT_3D('',#13841,#10900,#10901);
#9767=AXIS2_PLACEMENT_3D('',#13843,#10902,#10903);
#9768=AXIS2_PLACEMENT_3D('',#13846,#10905,#10906);
#9769=AXIS2_PLACEMENT_3D('',#13847,#10907,#10908);
#9770=AXIS2_PLACEMENT_3D('',#13849,#10909,#10910);
#9771=AXIS2_PLACEMENT_3D('',#13852,#10912,#10913);
#9772=AXIS2_PLACEMENT_3D('',#13853,#10914,#10915);
#9773=AXIS2_PLACEMENT_3D('',#13855,#10916,#10917);
#9774=AXIS2_PLACEMENT_3D('',#13858,#10919,#10920);
#9775=AXIS2_PLACEMENT_3D('',#13859,#10921,#10922);
#9776=AXIS2_PLACEMENT_3D('',#13861,#10923,#10924);
#9777=AXIS2_PLACEMENT_3D('',#13864,#10926,#10927);
#9778=AXIS2_PLACEMENT_3D('',#13865,#10928,#10929);
#9779=AXIS2_PLACEMENT_3D('',#13867,#10930,#10931);
#9780=AXIS2_PLACEMENT_3D('',#13870,#10933,#10934);
#9781=AXIS2_PLACEMENT_3D('',#13871,#10935,#10936);
#9782=AXIS2_PLACEMENT_3D('',#13873,#10937,#10938);
#9783=AXIS2_PLACEMENT_3D('',#13876,#10940,#10941);
#9784=AXIS2_PLACEMENT_3D('',#13877,#10942,#10943);
#9785=AXIS2_PLACEMENT_3D('',#13882,#10945,#10946);
#9786=AXIS2_PLACEMENT_3D('',#13886,#10949,#10950);
#9787=AXIS2_PLACEMENT_3D('',#13891,#10952,#10953);
#9788=AXIS2_PLACEMENT_3D('',#13895,#10956,#10957);
#9789=AXIS2_PLACEMENT_3D('',#13902,#10962,#10963);
#9790=AXIS2_PLACEMENT_3D('',#13911,#10968,#10969);
#9791=AXIS2_PLACEMENT_3D('',#13915,#10971,#10972);
#9792=AXIS2_PLACEMENT_3D('',#13919,#10975,#10976);
#9793=AXIS2_PLACEMENT_3D('',#13923,#10978,#10979);
#9794=AXIS2_PLACEMENT_3D('',#13927,#10982,#10983);
#9795=AXIS2_PLACEMENT_3D('',#13932,#10985,#10986);
#9796=AXIS2_PLACEMENT_3D('',#13935,#10988,#10989);
#9797=AXIS2_PLACEMENT_3D('',#13936,#10990,#10991);
#9798=AXIS2_PLACEMENT_3D('',#13942,#10995,#10996);
#9799=AXIS2_PLACEMENT_3D('',#13947,#10998,#10999);
#9800=AXIS2_PLACEMENT_3D('',#13950,#11001,#11002);
#9801=AXIS2_PLACEMENT_3D('',#13951,#11003,#11004);
#9802=AXIS2_PLACEMENT_3D('',#13957,#11008,#11009);
#9803=AXIS2_PLACEMENT_3D('',#13961,#11011,#11012);
#9804=AXIS2_PLACEMENT_3D('',#13962,#11013,#11014);
#9805=AXIS2_PLACEMENT_3D('',#13963,#11015,#11016);
#9806=AXIS2_PLACEMENT_3D('',#13969,#11020,#11021);
#9807=AXIS2_PLACEMENT_3D('',#13974,#11023,#11024);
#9808=AXIS2_PLACEMENT_3D('',#13977,#11026,#11027);
#9809=AXIS2_PLACEMENT_3D('',#13978,#11028,#11029);
#9810=AXIS2_PLACEMENT_3D('',#13981,#11032,#11033);
#9811=AXIS2_PLACEMENT_3D('',#13982,#11034,#11035);
#9812=AXIS2_PLACEMENT_3D('',#13983,#11036,#11037);
#9813=AXIS2_PLACEMENT_3D('',#13984,#11038,#11039);
#9814=AXIS2_PLACEMENT_3D('',#13988,#11041,#11042);
#9815=AXIS2_PLACEMENT_3D('',#13989,#11043,#11044);
#9816=AXIS2_PLACEMENT_3D('',#13990,#11045,#11046);
#9817=AXIS2_PLACEMENT_3D('',#13993,#11049,#11050);
#9818=AXIS2_PLACEMENT_3D('',#13997,#11052,#11053);
#9819=AXIS2_PLACEMENT_3D('',#13998,#11054,#11055);
#9820=AXIS2_PLACEMENT_3D('',#13999,#11056,#11057);
#9821=AXIS2_PLACEMENT_3D('',#14005,#11061,#11062);
#9822=AXIS2_PLACEMENT_3D('',#14007,#11063,#11064);
#9823=AXIS2_PLACEMENT_3D('',#14010,#11066,#11067);
#9824=AXIS2_PLACEMENT_3D('',#14011,#11068,#11069);
#9825=AXIS2_PLACEMENT_3D('',#14015,#11071,#11072);
#9826=AXIS2_PLACEMENT_3D('',#14016,#11073,#11074);
#9827=AXIS2_PLACEMENT_3D('',#14017,#11075,#11076);
#9828=AXIS2_PLACEMENT_3D('',#14023,#11080,#11081);
#9829=AXIS2_PLACEMENT_3D('',#14028,#11083,#11084);
#9830=AXIS2_PLACEMENT_3D('',#14031,#11086,#11087);
#9831=AXIS2_PLACEMENT_3D('',#14032,#11088,#11089);
#9832=AXIS2_PLACEMENT_3D('',#14035,#11092,#11093);
#9833=AXIS2_PLACEMENT_3D('',#14040,#11097,#11098);
#9834=AXIS2_PLACEMENT_3D('',#14044,#11101,#11102);
#9835=AXIS2_PLACEMENT_3D('',#14047,#11105,#11106);
#9836=AXIS2_PLACEMENT_3D('',#14049,#11108,#11109);
#9837=AXIS2_PLACEMENT_3D('',#14051,#11111,#11112);
#9838=AXIS2_PLACEMENT_3D('',#14052,#11113,#11114);
#9839=AXIS2_PLACEMENT_3D('',#14054,#11116,#11117);
#9840=AXIS2_PLACEMENT_3D('',#14056,#11119,#11120);
#9841=AXIS2_PLACEMENT_3D('',#14058,#11122,#11123);
#9842=AXIS2_PLACEMENT_3D('',#14060,#11125,#11126);
#9843=AXIS2_PLACEMENT_3D('',#14062,#11128,#11129);
#9844=AXIS2_PLACEMENT_3D('',#14066,#11132,#11133);
#9845=AXIS2_PLACEMENT_3D('',#14070,#11136,#11137);
#9846=AXIS2_PLACEMENT_3D('',#14073,#11140,#11141);
#9847=AXIS2_PLACEMENT_3D('',#14075,#11143,#11144);
#9848=AXIS2_PLACEMENT_3D('',#14077,#11146,#11147);
#9849=AXIS2_PLACEMENT_3D('',#14079,#11149,#11150);
#9850=AXIS2_PLACEMENT_3D('',#14081,#11152,#11153);
#9851=AXIS2_PLACEMENT_3D('',#14084,#11156,#11157);
#9852=AXIS2_PLACEMENT_3D('',#14088,#11161,#11162);
#9853=AXIS2_PLACEMENT_3D('',#14090,#11164,#11165);
#9854=AXIS2_PLACEMENT_3D('',#14091,#11166,#11167);
#9855=AXIS2_PLACEMENT_3D('',#14092,#11168,#11169);
#9856=AXIS2_PLACEMENT_3D('',#14093,#11170,#11171);
#9857=AXIS2_PLACEMENT_3D('',#14095,#11172,#11173);
#9858=AXIS2_PLACEMENT_3D('',#14098,#11175,#11176);
#9859=AXIS2_PLACEMENT_3D('',#14099,#11177,#11178);
#9860=AXIS2_PLACEMENT_3D('',#14101,#11179,#11180);
#9861=AXIS2_PLACEMENT_3D('',#14103,#11181,#11182);
#9862=AXIS2_PLACEMENT_3D('',#14105,#11184,#11185);
#9863=AXIS2_PLACEMENT_3D('',#14107,#11187,#11188);
#9864=AXIS2_PLACEMENT_3D('',#14109,#11190,#11191);
#9865=AXIS2_PLACEMENT_3D('',#14115,#11195,#11196);
#9866=AXIS2_PLACEMENT_3D('',#14121,#11200,#11201);
#9867=AXIS2_PLACEMENT_3D('',#14127,#11205,#11206);
#9868=AXIS2_PLACEMENT_3D('',#14133,#11210,#11211);
#9869=AXIS2_PLACEMENT_3D('',#14135,#11213,#11214);
#9870=AXIS2_PLACEMENT_3D('',#14137,#11216,#11217);
#9871=AXIS2_PLACEMENT_3D('',#14138,#11218,#11219);
#9872=AXIS2_PLACEMENT_3D('',#14140,#11220,#11221);
#9873=AXIS2_PLACEMENT_3D('',#14142,#11222,#11223);
#9874=AXIS2_PLACEMENT_3D('',#14144,#11225,#11226);
#9875=AXIS2_PLACEMENT_3D('',#14146,#11227,#11228);
#9876=AXIS2_PLACEMENT_3D('',#14148,#11229,#11230);
#9877=AXIS2_PLACEMENT_3D('',#14150,#11232,#11233);
#9878=AXIS2_PLACEMENT_3D('',#14152,#11235,#11236);
#9879=AXIS2_PLACEMENT_3D('',#14154,#11238,#11239);
#9880=AXIS2_PLACEMENT_3D('',#14160,#11243,#11244);
#9881=AXIS2_PLACEMENT_3D('',#14166,#11248,#11249);
#9882=AXIS2_PLACEMENT_3D('',#14172,#11253,#11254);
#9883=AXIS2_PLACEMENT_3D('',#14178,#11258,#11259);
#9884=AXIS2_PLACEMENT_3D('',#14180,#11261,#11262);
#9885=AXIS2_PLACEMENT_3D('',#14182,#11264,#11265);
#10863=DIRECTION('axis',(0.,0.,1.));
#10864=DIRECTION('refdir',(1.,0.,0.));
#10865=DIRECTION('center_axis',(1.,3.89551938464967E-15,6.32781493568956E-31));
#10866=DIRECTION('ref_axis',(-3.89551938464967E-15,1.,8.11109567411167E-62));
#10867=DIRECTION('center_axis',(-1.,-3.89551938464967E-15,-6.32181852599599E-31));
#10868=DIRECTION('ref_axis',(3.89551938464967E-15,-1.,2.46267666142548E-45));
#10869=DIRECTION('',(1.,3.89551938464967E-15,6.32781493568956E-31));
#10870=DIRECTION('center_axis',(1.,3.89551938464967E-15,6.32781493568956E-31));
#10871=DIRECTION('ref_axis',(-3.89551938464967E-15,1.,-2.46501257444544E-45));
#10872=DIRECTION('center_axis',(1.,3.89551938464967E-15,6.32781493568956E-31));
#10873=DIRECTION('ref_axis',(-3.89551938464967E-15,1.,-4.58615050165474E-60));
#10874=DIRECTION('center_axis',(-1.,-3.89551938464967E-15,-6.32181852599599E-31));
#10875=DIRECTION('ref_axis',(3.89551938464967E-15,-1.,2.46267666142548E-45));
#10876=DIRECTION('',(1.,3.89551938464967E-15,6.32781493568956E-31));
#10877=DIRECTION('center_axis',(1.,3.89551938464967E-15,6.32781493568956E-31));
#10878=DIRECTION('ref_axis',(-3.89551938464967E-15,1.,-2.46501257444544E-45));
#10879=DIRECTION('center_axis',(1.,3.89551938464967E-15,6.32781493568956E-31));
#10880=DIRECTION('ref_axis',(-3.89551938464967E-15,1.,8.11109567411167E-62));
#10881=DIRECTION('center_axis',(1.,3.89551938464967E-15,6.32781493568956E-31));
#10882=DIRECTION('ref_axis',(-3.89551938464967E-15,1.,1.11134276064131E-61));
#10883=DIRECTION('',(1.,3.89551938464967E-15,6.32781493568956E-31));
#10884=DIRECTION('center_axis',(1.,-3.49148133884313E-15,-5.66612798746291E-31));
#10885=DIRECTION('ref_axis',(3.49148133884313E-15,1.,-1.24849656241355E-47));
#10886=DIRECTION('center_axis',(1.,3.89551938464967E-15,6.32781493568956E-31));
#10887=DIRECTION('ref_axis',(-3.89551938464967E-15,1.,-4.58615050165474E-60));
#10888=DIRECTION('center_axis',(1.,3.89551938464967E-15,6.32781493568956E-31));
#10889=DIRECTION('ref_axis',(-3.89551938464967E-15,1.,-4.55612718233173E-60));
#10890=DIRECTION('',(1.,3.89551938464967E-15,6.32781493568956E-31));
#10891=DIRECTION('center_axis',(1.,-3.49148133884313E-15,-5.66612798746291E-31));
#10892=DIRECTION('ref_axis',(3.49148133884313E-15,1.,-1.24849656241308E-47));
#10893=DIRECTION('center_axis',(0.,-1.,-1.22464679914735E-16));
#10894=DIRECTION('ref_axis',(0.,1.22464679914735E-16,-1.));
#10895=DIRECTION('center_axis',(0.,-1.,-1.22464679914735E-16));
#10896=DIRECTION('ref_axis',(0.,1.22464679914735E-16,-1.));
#10897=DIRECTION('',(0.,-1.,-1.22464679914735E-16));
#10898=DIRECTION('center_axis',(0.,-1.,-1.22464679914735E-16));
#10899=DIRECTION('ref_axis',(0.,1.22464679914735E-16,-1.));
#10900=DIRECTION('center_axis',(0.,-1.,-1.22464679914735E-16));
#10901=DIRECTION('ref_axis',(0.,1.22464679914735E-16,-1.));
#10902=DIRECTION('center_axis',(0.,-1.,-1.22464679914735E-16));
#10903=DIRECTION('ref_axis',(0.,1.22464679914735E-16,-1.));
#10904=DIRECTION('',(0.,-1.,-1.22464679914735E-16));
#10905=DIRECTION('center_axis',(0.,-1.,-1.22464679914735E-16));
#10906=DIRECTION('ref_axis',(0.,1.22464679914735E-16,-1.));
#10907=DIRECTION('center_axis',(0.,-1.,-1.22464679914735E-16));
#10908=DIRECTION('ref_axis',(0.,1.22464679914735E-16,-1.));
#10909=DIRECTION('center_axis',(0.,-1.,0.));
#10910=DIRECTION('ref_axis',(0.,0.,-1.));
#10911=DIRECTION('',(0.,-1.,-1.22464679914735E-16));
#10912=DIRECTION('center_axis',(0.,-1.,-1.22464679914735E-16));
#10913=DIRECTION('ref_axis',(0.,1.22464679914735E-16,-1.));
#10914=DIRECTION('center_axis',(0.,-1.,0.));
#10915=DIRECTION('ref_axis',(0.,0.,-1.));
#10916=DIRECTION('center_axis',(0.,-1.,-1.22464679914735E-16));
#10917=DIRECTION('ref_axis',(0.,1.22464679914735E-16,-1.));
#10918=DIRECTION('',(0.,-1.,0.));
#10919=DIRECTION('center_axis',(0.,-1.,0.));
#10920=DIRECTION('ref_axis',(0.,0.,1.));
#10921=DIRECTION('center_axis',(0.,-1.,0.));
#10922=DIRECTION('ref_axis',(0.,0.,-1.));
#10923=DIRECTION('center_axis',(0.,-1.,-1.22464679914735E-16));
#10924=DIRECTION('ref_axis',(0.,1.22464679914735E-16,-1.));
#10925=DIRECTION('',(0.,-1.,0.));
#10926=DIRECTION('center_axis',(0.,-1.,0.));
#10927=DIRECTION('ref_axis',(0.,0.,-1.));
#10928=DIRECTION('center_axis',(0.,-1.,0.));
#10929=DIRECTION('ref_axis',(0.,0.,-1.));
#10930=DIRECTION('center_axis',(0.,-1.,0.));
#10931=DIRECTION('ref_axis',(0.,0.,-1.));
#10932=DIRECTION('',(0.,-1.,0.));
#10933=DIRECTION('center_axis',(0.,-1.,0.));
#10934=DIRECTION('ref_axis',(0.,0.,1.));
#10935=DIRECTION('center_axis',(0.,-1.,0.));
#10936=DIRECTION('ref_axis',(0.,0.,-1.));
#10937=DIRECTION('center_axis',(0.,-1.,0.));
#10938=DIRECTION('ref_axis',(0.,0.,-1.));
#10939=DIRECTION('',(0.,-1.,0.));
#10940=DIRECTION('center_axis',(0.,-1.,0.));
#10941=DIRECTION('ref_axis',(0.,0.,-1.));
#10942=DIRECTION('center_axis',(1.0842021724855E-15,-6.12323399573677E-17,
1.));
#10943=DIRECTION('ref_axis',(1.,-2.72542236090223E-48,-1.0842021724855E-15));
#10944=DIRECTION('',(1.,0.,-1.08420217248551E-15));
#10945=DIRECTION('center_axis',(0.,0.,-1.));
#10946=DIRECTION('ref_axis',(-1.,0.,0.));
#10947=DIRECTION('',(1.,0.,0.));
#10948=DIRECTION('',(0.,-1.,-2.89120579329468E-16));
#10949=DIRECTION('center_axis',(-4.24884710452154E-31,6.12323399573677E-17,
-1.));
#10950=DIRECTION('ref_axis',(0.,1.,6.12323399573677E-17));
#10951=DIRECTION('',(-1.,0.,0.));
#10952=DIRECTION('center_axis',(0.,0.,1.));
#10953=DIRECTION('ref_axis',(-1.,0.,0.));
#10954=DIRECTION('',(-1.,-6.93889390390723E-15,0.));
#10955=DIRECTION('',(0.,1.,0.));
#10956=DIRECTION('center_axis',(0.,1.,1.5770213417971E-16));
#10957=DIRECTION('ref_axis',(0.,-1.5770213417971E-16,1.));
#10958=DIRECTION('',(-1.,0.,0.));
#10959=DIRECTION('',(0.,0.,1.));
#10960=DIRECTION('',(-1.,0.,0.));
#10961=DIRECTION('',(0.,0.,-1.));
#10962=DIRECTION('center_axis',(0.,1.,1.5770213417971E-16));
#10963=DIRECTION('ref_axis',(0.,-1.5770213417971E-16,1.));
#10964=DIRECTION('',(0.,0.,1.));
#10965=DIRECTION('',(-1.,0.,0.));
#10966=DIRECTION('',(0.,0.,-1.));
#10967=DIRECTION('',(-1.,0.,0.));
#10968=DIRECTION('center_axis',(-4.24884710452153E-31,6.12323399573677E-17,
-1.));
#10969=DIRECTION('ref_axis',(0.,1.,6.12323399573677E-17));
#10970=DIRECTION('',(-1.,0.,0.));
#10971=DIRECTION('center_axis',(0.,0.,1.));
#10972=DIRECTION('ref_axis',(1.,0.,0.));
#10973=DIRECTION('',(-1.,0.,0.));
#10974=DIRECTION('',(0.,-1.,0.));
#10975=DIRECTION('center_axis',(8.67361737988404E-16,-6.12323399573677E-17,
1.));
#10976=DIRECTION('ref_axis',(1.,5.37018253511908E-48,-8.67361737988404E-16));
#10977=DIRECTION('',(-1.,0.,0.));
#10978=DIRECTION('center_axis',(0.,0.,-1.));
#10979=DIRECTION('ref_axis',(1.,-2.42861286636753E-14,0.));
#10980=DIRECTION('',(-1.,0.,0.));
#10981=DIRECTION('',(0.,1.,2.89120579329468E-16));
#10982=DIRECTION('center_axis',(1.,0.,0.));
#10983=DIRECTION('ref_axis',(0.,0.,-1.));
#10984=DIRECTION('',(0.,0.,-1.));
#10985=DIRECTION('center_axis',(-1.,0.,0.));
#10986=DIRECTION('ref_axis',(0.,0.,-1.));
#10987=DIRECTION('',(0.,-1.,0.));
#10988=DIRECTION('center_axis',(-1.,0.,0.));
#10989=DIRECTION('ref_axis',(0.,0.,-1.));
#10990=DIRECTION('center_axis',(1.,0.,0.));
#10991=DIRECTION('ref_axis',(0.,0.,-1.));
#10992=DIRECTION('',(0.,1.,0.));
#10993=DIRECTION('',(0.,1.,0.));
#10994=DIRECTION('',(0.,0.,1.));
#10995=DIRECTION('center_axis',(-1.,0.,0.));
#10996=DIRECTION('ref_axis',(0.,0.,1.));
#10997=DIRECTION('',(0.,1.,0.));
#10998=DIRECTION('center_axis',(-1.,0.,0.));
#10999=DIRECTION('ref_axis',(0.,0.,-1.));
#11000=DIRECTION('',(0.,0.,1.));
#11001=DIRECTION('center_axis',(-1.,0.,0.));
#11002=DIRECTION('ref_axis',(0.,0.,-1.));
#11003=DIRECTION('center_axis',(-1.,0.,0.));
#11004=DIRECTION('ref_axis',(0.,0.,1.));
#11005=DIRECTION('',(0.,0.,1.));
#11006=DIRECTION('',(0.,0.,1.));
#11007=DIRECTION('',(0.,-1.,0.));
#11008=DIRECTION('center_axis',(1.,0.,0.));
#11009=DIRECTION('ref_axis',(0.,0.,-1.));
#11010=DIRECTION('',(0.,-0.889029388585715,-0.457850135121645));
#11011=DIRECTION('center_axis',(-1.,0.,0.));
#11012=DIRECTION('ref_axis',(0.,-6.93889390390722E-15,-1.));
#11013=DIRECTION('center_axis',(-1.,0.,0.));
#11014=DIRECTION('ref_axis',(0.,-2.08166817117217E-14,-1.));
#11015=DIRECTION('center_axis',(1.,0.,0.));
#11016=DIRECTION('ref_axis',(0.,0.,-1.));
#11017=DIRECTION('',(0.,0.457850135121644,-0.889029388585716));
#11018=DIRECTION('',(0.,0.457850135121643,-0.889029388585717));
#11019=DIRECTION('',(0.,0.889029388585714,0.457850135121648));
#11020=DIRECTION('center_axis',(-1.,0.,0.));
#11021=DIRECTION('ref_axis',(0.,0.,1.));
#11022=DIRECTION('',(0.,0.,-1.));
#11023=DIRECTION('center_axis',(-1.,0.,0.));
#11024=DIRECTION('ref_axis',(0.,-6.93889390390722E-15,-1.));
#11025=DIRECTION('',(0.,0.889029388585715,0.457850135121645));
#11026=DIRECTION('center_axis',(-1.,0.,0.));
#11027=DIRECTION('ref_axis',(0.,-2.08166817117217E-14,-1.));
#11028=DIRECTION('center_axis',(-1.,0.,0.));
#11029=DIRECTION('ref_axis',(0.,0.,1.));
#11030=DIRECTION('',(0.,1.,0.));
#11031=DIRECTION('',(0.,1.,0.));
#11032=DIRECTION('center_axis',(1.,0.,0.));
#11033=DIRECTION('ref_axis',(0.,0.,-1.));
#11034=DIRECTION('center_axis',(-1.,0.,0.));
#11035=DIRECTION('ref_axis',(0.,1.73472347597681E-14,-1.));
#11036=DIRECTION('center_axis',(-1.,0.,0.));
#11037=DIRECTION('ref_axis',(0.,0.,-1.));
#11038=DIRECTION('center_axis',(-1.,0.,0.));
#11039=DIRECTION('ref_axis',(0.,0.,1.));
#11040=DIRECTION('',(0.,-0.889029388585714,-0.457850135121648));
#11041=DIRECTION('center_axis',(-1.,0.,0.));
#11042=DIRECTION('ref_axis',(0.,1.73472347597681E-14,-1.));
#11043=DIRECTION('center_axis',(-1.,0.,0.));
#11044=DIRECTION('ref_axis',(0.,0.,-1.));
#11045=DIRECTION('center_axis',(-1.,0.,0.));
#11046=DIRECTION('ref_axis',(0.,0.,1.));
#11047=DIRECTION('',(0.,0.457850135121644,-0.889029388585716));
#11048=DIRECTION('',(0.,0.457850135121643,-0.889029388585717));
#11049=DIRECTION('center_axis',(1.,0.,0.));
#11050=DIRECTION('ref_axis',(0.,0.,-1.));
#11051=DIRECTION('',(0.,0.,1.));
#11052=DIRECTION('center_axis',(-1.,0.,0.));
#11053=DIRECTION('ref_axis',(0.,0.,-1.));
#11054=DIRECTION('center_axis',(-1.,0.,0.));
#11055=DIRECTION('ref_axis',(0.,0.,-1.));
#11056=DIRECTION('center_axis',(1.,0.,0.));
#11057=DIRECTION('ref_axis',(0.,0.,-1.));
#11058=DIRECTION('',(0.,-1.,0.));
#11059=DIRECTION('',(0.,-1.,0.));
#11060=DIRECTION('',(0.,0.,-1.));
#11061=DIRECTION('center_axis',(-1.,0.,0.));
#11062=DIRECTION('ref_axis',(0.,0.,1.));
#11063=DIRECTION('center_axis',(-1.,0.,0.));
#11064=DIRECTION('ref_axis',(0.,0.,-1.));
#11065=DIRECTION('',(0.,0.,-1.));
#11066=DIRECTION('center_axis',(-1.,0.,0.));
#11067=DIRECTION('ref_axis',(0.,0.,-1.));
#11068=DIRECTION('center_axis',(1.,0.,0.));
#11069=DIRECTION('ref_axis',(0.,0.,-1.));
#11070=DIRECTION('',(0.,1.,0.));
#11071=DIRECTION('center_axis',(-1.,0.,0.));
#11072=DIRECTION('ref_axis',(0.,0.,-1.));
#11073=DIRECTION('center_axis',(-1.,0.,0.));
#11074=DIRECTION('ref_axis',(0.,0.,-1.));
#11075=DIRECTION('center_axis',(1.,0.,0.));
#11076=DIRECTION('ref_axis',(0.,0.,-1.));
#11077=DIRECTION('',(0.,-1.22464679914735E-16,1.));
#11078=DIRECTION('',(0.,-1.22464679914735E-16,1.));
#11079=DIRECTION('',(0.,1.,0.));
#11080=DIRECTION('center_axis',(-1.,0.,0.));
#11081=DIRECTION('ref_axis',(0.,0.,1.));
#11082=DIRECTION('',(0.,0.,1.));
#11083=DIRECTION('center_axis',(-1.,0.,0.));
#11084=DIRECTION('ref_axis',(0.,0.,-1.));
#11085=DIRECTION('',(0.,-1.,0.));
#11086=DIRECTION('center_axis',(-1.,0.,0.));
#11087=DIRECTION('ref_axis',(0.,0.,-1.));
#11088=DIRECTION('center_axis',(-1.,0.,0.));
#11089=DIRECTION('ref_axis',(0.,0.,1.));
#11090=DIRECTION('',(0.,-1.,0.));
#11091=DIRECTION('',(0.,-1.,0.));
#11092=DIRECTION('center_axis',(0.,-1.,-1.22464679914735E-16));
#11093=DIRECTION('ref_axis',(0.,1.22464679914735E-16,-1.));
#11094=DIRECTION('',(0.,-1.22464679914735E-16,1.));
#11095=DIRECTION('',(-1.,0.,0.));
#11096=DIRECTION('',(-1.,0.,0.));
#11097=DIRECTION('center_axis',(0.,0.,1.));
#11098=DIRECTION('ref_axis',(1.,0.,0.));
#11099=DIRECTION('',(0.,1.,0.));
#11100=DIRECTION('',(-1.,0.,0.));
#11101=DIRECTION('center_axis',(0.,-1.,-1.22464679914735E-16));
#11102=DIRECTION('ref_axis',(0.,1.22464679914735E-16,-1.));
#11103=DIRECTION('',(0.,-1.22464679914735E-16,1.));
#11104=DIRECTION('',(-1.,0.,0.));
#11105=DIRECTION('center_axis',(-1.,0.,0.));
#11106=DIRECTION('ref_axis',(0.,0.,1.));
#11107=DIRECTION('',(-1.,0.,0.));
#11108=DIRECTION('center_axis',(0.,0.,-1.));
#11109=DIRECTION('ref_axis',(-1.,0.,0.));
#11110=DIRECTION('',(-1.,0.,0.));
#11111=DIRECTION('center_axis',(-1.,0.,0.));
#11112=DIRECTION('ref_axis',(0.,0.,1.));
#11113=DIRECTION('center_axis',(-1.,0.,0.));
#11114=DIRECTION('ref_axis',(0.,0.,1.));
#11115=DIRECTION('',(-1.,0.,0.));
#11116=DIRECTION('center_axis',(0.,0.889029388585716,0.457850135121643));
#11117=DIRECTION('ref_axis',(0.,-0.457850135121643,0.889029388585716));
#11118=DIRECTION('',(-1.,0.,0.));
#11119=DIRECTION('center_axis',(-1.,0.,0.));
#11120=DIRECTION('ref_axis',(0.,0.,1.));
#11121=DIRECTION('',(-1.,0.,0.));
#11122=DIRECTION('center_axis',(0.,0.,1.));
#11123=DIRECTION('ref_axis',(1.,0.,0.));
#11124=DIRECTION('',(-1.,0.,0.));
#11125=DIRECTION('center_axis',(-1.,0.,0.));
#11126=DIRECTION('ref_axis',(0.,0.,1.));
#11127=DIRECTION('',(-1.,0.,0.));
#11128=DIRECTION('center_axis',(0.,-1.,0.));
#11129=DIRECTION('ref_axis',(0.,0.,-1.));
#11130=DIRECTION('',(-1.,0.,0.));
#11131=DIRECTION('',(0.,0.,1.));
#11132=DIRECTION('center_axis',(0.,0.,-1.));
#11133=DIRECTION('ref_axis',(-1.,0.,0.));
#11134=DIRECTION('',(-1.,0.,0.));
#11135=DIRECTION('',(0.,-1.,0.));
#11136=DIRECTION('center_axis',(0.,-1.,0.));
#11137=DIRECTION('ref_axis',(0.,0.,-1.));
#11138=DIRECTION('',(-1.,0.,0.));
#11139=DIRECTION('',(0.,0.,1.));
#11140=DIRECTION('center_axis',(-1.,0.,0.));
#11141=DIRECTION('ref_axis',(0.,0.,1.));
#11142=DIRECTION('',(-1.,0.,0.));
#11143=DIRECTION('center_axis',(0.,0.,1.));
#11144=DIRECTION('ref_axis',(1.,0.,0.));
#11145=DIRECTION('',(-1.,0.,0.));
#11146=DIRECTION('center_axis',(-1.,0.,0.));
#11147=DIRECTION('ref_axis',(0.,0.,1.));
#11148=DIRECTION('',(-1.,0.,0.));
#11149=DIRECTION('center_axis',(0.,0.889029388585716,0.457850135121643));
#11150=DIRECTION('ref_axis',(0.,-0.457850135121644,0.889029388585716));
#11151=DIRECTION('',(-1.,0.,0.));
#11152=DIRECTION('center_axis',(-1.,0.,0.));
#11153=DIRECTION('ref_axis',(0.,0.,1.));
#11154=DIRECTION('',(-1.,-6.93889390390723E-15,0.));
#11155=DIRECTION('',(-1.,0.,0.));
#11156=DIRECTION('center_axis',(-1.,0.,0.));
#11157=DIRECTION('ref_axis',(0.,0.,1.));
#11158=DIRECTION('',(-1.,0.,0.));
#11159=DIRECTION('',(-1.,0.,0.));
#11160=DIRECTION('',(1.,0.,-1.08420217248551E-15));
#11161=DIRECTION('center_axis',(0.,0.,-1.));
#11162=DIRECTION('ref_axis',(-1.,0.,0.));
#11163=DIRECTION('',(-1.,0.,0.));
#11164=DIRECTION('center_axis',(-1.,0.,0.));
#11165=DIRECTION('ref_axis',(0.,0.,1.));
#11166=DIRECTION('center_axis',(1.,0.,0.));
#11167=DIRECTION('ref_axis',(0.,0.,-1.));
#11168=DIRECTION('center_axis',(1.,0.,0.));
#11169=DIRECTION('ref_axis',(0.,0.,-1.));
#11170=DIRECTION('center_axis',(0.,0.,-1.));
#11171=DIRECTION('ref_axis',(-1.,0.,0.));
#11172=DIRECTION('center_axis',(0.,0.,-1.));
#11173=DIRECTION('ref_axis',(1.,1.76941794549634E-13,0.));
#11174=DIRECTION('',(1.,3.89551938464967E-15,6.46539339818476E-31));
#11175=DIRECTION('center_axis',(0.,0.,-1.));
#11176=DIRECTION('ref_axis',(1.,0.,0.));
#11177=DIRECTION('center_axis',(0.,0.,-1.));
#11178=DIRECTION('ref_axis',(-1.,0.,0.));
#11179=DIRECTION('center_axis',(0.,0.,1.));
#11180=DIRECTION('ref_axis',(1.,0.,0.));
#11181=DIRECTION('center_axis',(0.,0.,1.));
#11182=DIRECTION('ref_axis',(1.,0.,0.));
#11183=DIRECTION('',(1.,3.89551938464967E-15,5.66612798746291E-31));
#11184=DIRECTION('center_axis',(0.,0.,1.));
#11185=DIRECTION('ref_axis',(1.,3.46944695195361E-15,0.));
#11186=DIRECTION('',(6.32181852599599E-31,2.46267666142548E-45,-1.));
#11187=DIRECTION('center_axis',(0.,0.,1.));
#11188=DIRECTION('ref_axis',(1.,0.,0.));
#11189=DIRECTION('',(-6.32181852599599E-31,-2.46267666142548E-45,1.));
#11190=DIRECTION('center_axis',(5.66612798746291E-31,2.20725114110678E-45,
-1.));
#11191=DIRECTION('ref_axis',(-1.,1.16909086576945E-91,-5.66612798746291E-31));
#11192=DIRECTION('',(3.89551938464967E-15,-1.,0.));
#11193=DIRECTION('',(1.,3.89551938464967E-15,6.32781493568956E-31));
#11194=DIRECTION('',(3.89551938464967E-15,-1.,0.));
#11195=DIRECTION('center_axis',(1.24069748425108E-31,-1.97819343751741E-16,
1.));
#11196=DIRECTION('ref_axis',(0.,-1.,-1.97819343751741E-16));
#11197=DIRECTION('',(-3.89551938464967E-15,1.,1.97819343751741E-16));
#11198=DIRECTION('',(-1.,-3.49148133884313E-15,-5.66612798746291E-31));
#11199=DIRECTION('',(-3.89551938464967E-15,1.,1.97819343751741E-16));
#11200=DIRECTION('center_axis',(-1.,-3.89551938464967E-15,-6.32181852599599E-31));
#11201=DIRECTION('ref_axis',(3.89551938464967E-15,-1.,3.65599846003365E-62));
#11202=DIRECTION('',(1.84901925624628E-15,-0.450343689478977,0.892855285780659));
#11203=DIRECTION('',(4.27488727659472E-15,-1.,0.));
#11204=DIRECTION('',(8.75811540203011E-47,1.62284355480483E-16,-1.));
#11205=DIRECTION('center_axis',(-1.,-3.89551938464967E-15,-6.32181852599599E-31));
#11206=DIRECTION('ref_axis',(3.89551938464967E-15,-1.,3.65599846003365E-62));
#11207=DIRECTION('',(8.75811540203011E-47,1.62284355480483E-16,-1.));
#11208=DIRECTION('',(4.27488727659472E-15,-1.,0.));
#11209=DIRECTION('',(1.84901925624628E-15,-0.450343689478977,0.892855285780659));
#11210=DIRECTION('center_axis',(-3.49148133884313E-15,1.,1.62284355480483E-16));
#11211=DIRECTION('ref_axis',(-1.,-3.49148133884313E-15,0.));
#11212=DIRECTION('',(1.,3.89551938464967E-15,6.32781493568956E-31));
#11213=DIRECTION('center_axis',(-6.32781493568956E-31,-2.70506955572254E-45,
1.));
#11214=DIRECTION('ref_axis',(1.,-7.97759856789153E-92,6.32781493568956E-31));
#11215=DIRECTION('',(1.,3.89551938464967E-15,6.32781493568956E-31));
#11216=DIRECTION('center_axis',(-3.47813507344548E-15,0.892855285780659,
0.450343689478978));
#11217=DIRECTION('ref_axis',(5.27827569634311E-32,-0.450343689478977,0.892855285780659));
#11218=DIRECTION('center_axis',(0.,0.,1.));
#11219=DIRECTION('ref_axis',(1.,0.,0.));
#11220=DIRECTION('center_axis',(0.,0.,1.));
#11221=DIRECTION('ref_axis',(-1.,0.,0.));
#11222=DIRECTION('center_axis',(0.,0.,1.));
#11223=DIRECTION('ref_axis',(-1.,3.46944695195361E-15,0.));
#11224=DIRECTION('',(-1.,3.49148133884313E-15,5.66612798746291E-31));
#11225=DIRECTION('center_axis',(0.,0.,1.));
#11226=DIRECTION('ref_axis',(1.,0.,0.));
#11227=DIRECTION('center_axis',(0.,0.,-1.));
#11228=DIRECTION('ref_axis',(-1.,0.,0.));
#11229=DIRECTION('center_axis',(0.,0.,-1.));
#11230=DIRECTION('ref_axis',(-1.,0.,0.));
#11231=DIRECTION('',(-1.,3.49148133884313E-15,5.66612798746291E-31));
#11232=DIRECTION('center_axis',(0.,0.,-1.));
#11233=DIRECTION('ref_axis',(-1.,3.46944695195361E-15,0.));
#11234=DIRECTION('',(0.,-1.62284355480483E-16,1.));
#11235=DIRECTION('center_axis',(0.,0.,-1.));
#11236=DIRECTION('ref_axis',(-1.,0.,0.));
#11237=DIRECTION('',(0.,1.62284355480483E-16,-1.));
#11238=DIRECTION('center_axis',(-5.66612798746291E-31,1.97831801317236E-45,
-1.));
#11239=DIRECTION('ref_axis',(-1.,3.87718526908309E-92,5.66612798746291E-31));
#11240=DIRECTION('',(3.49148133884313E-15,1.,0.));
#11241=DIRECTION('',(-1.,3.49148133884313E-15,5.6715024575856E-31));
#11242=DIRECTION('',(3.49148133884313E-15,1.,0.));
#11243=DIRECTION('center_axis',(-7.61622868891015E-31,-3.80421814907195E-16,
1.));
#11244=DIRECTION('ref_axis',(0.,-1.,-3.80421814907195E-16));
#11245=DIRECTION('',(-3.49148133884313E-15,-1.,-3.80421814907195E-16));
#11246=DIRECTION('',(1.,-3.49148133884313E-15,-5.66612798746291E-31));
#11247=DIRECTION('',(-3.49148133884313E-15,-1.,-3.80421814907195E-16));
#11248=DIRECTION('center_axis',(1.,-3.49148133884313E-15,-5.66612798746291E-31));
#11249=DIRECTION('ref_axis',(3.49148133884313E-15,1.,-3.25324957840726E-62));
#11250=DIRECTION('',(0.,-1.62284355480483E-16,1.));
#11251=DIRECTION('',(3.49148133884313E-15,1.,0.));
#11252=DIRECTION('',(1.57236658788162E-15,0.450343689478977,-0.892855285780659));
#11253=DIRECTION('center_axis',(1.,-3.49148133884313E-15,-5.66612798746291E-31));
#11254=DIRECTION('ref_axis',(3.49148133884313E-15,1.,-3.25324957840726E-62));
#11255=DIRECTION('',(1.57236658788162E-15,0.450343689478977,-0.892855285780659));
#11256=DIRECTION('',(3.49148133884313E-15,1.,0.));
#11257=DIRECTION('',(0.,-1.62284355480483E-16,1.));
#11258=DIRECTION('center_axis',(3.49148133884313E-15,1.,1.62284355480483E-16));
#11259=DIRECTION('ref_axis',(-1.,3.49148133884313E-15,0.));
#11260=DIRECTION('',(-1.,3.49148133884313E-15,5.6715024575856E-31));
#11261=DIRECTION('center_axis',(3.11738756859062E-15,0.892855285780659,
0.450343689478978));
#11262=DIRECTION('ref_axis',(6.19177544941703E-32,-0.450343689478977,0.892855285780659));
#11263=DIRECTION('',(-1.,3.49148133884313E-15,5.6715024575856E-31));
#11264=DIRECTION('center_axis',(5.6715024575856E-31,-1.98019449938631E-45,
1.));
#11265=DIRECTION('ref_axis',(1.,8.02907465960574E-92,-5.6715024575856E-31));
#13810=CARTESIAN_POINT('',(0.,0.,0.));
#13811=CARTESIAN_POINT('Origin',(-4.44089209850063E-13,37.83598559535,138.));
#13812=CARTESIAN_POINT('',(682.31,31.8359855953526,138.));
#13813=CARTESIAN_POINT('Origin',(682.31,37.8359855953526,138.));
#13814=CARTESIAN_POINT('',(685.31,31.8359855953526,138.));
#13815=CARTESIAN_POINT('',(-4.20716093542164E-13,31.83598559535,138.));
#13816=CARTESIAN_POINT('Origin',(685.31,37.8359855953527,138.));
#13817=CARTESIAN_POINT('Origin',(-4.44089209850063E-13,35.9826602645986,
63.0000000000002));
#13818=CARTESIAN_POINT('',(682.31,29.9826602646013,63.0000000000002));
#13819=CARTESIAN_POINT('Origin',(682.31,35.9826602646013,63.0000000000002));
#13820=CARTESIAN_POINT('',(685.31,29.9826602646013,63.0000000000002));
#13821=CARTESIAN_POINT('',(-4.20716093542165E-13,29.9826602645986,63.0000000000002));
#13822=CARTESIAN_POINT('Origin',(685.31,35.9826602646013,63.0000000000002));
#13823=CARTESIAN_POINT('Origin',(-4.44089209850063E-13,37.83598559535,138.));
#13824=CARTESIAN_POINT('',(-4.20716093542164E-13,31.83598559535,138.));
#13825=CARTESIAN_POINT('Origin',(-4.44089209850063E-13,37.83598559535,138.));
#13826=CARTESIAN_POINT('',(2.99999999999997,31.83598559535,138.));
#13827=CARTESIAN_POINT('',(-4.20716093542164E-13,31.83598559535,138.));
#13828=CARTESIAN_POINT('Origin',(2.9999999999999,37.83598559535,138.));
#13829=CARTESIAN_POINT('Origin',(-4.44089209850063E-13,35.9826602645986,
63.0000000000002));
#13830=CARTESIAN_POINT('',(-4.20716093542165E-13,29.9826602645986,63.0000000000002));
#13831=CARTESIAN_POINT('Origin',(-4.44089209850063E-13,35.9826602645986,
63.0000000000002));
#13832=CARTESIAN_POINT('',(2.99999999999996,29.9826602645986,63.0000000000002));
#13833=CARTESIAN_POINT('',(-4.20716093542165E-13,29.9826602645986,63.0000000000002));
#13834=CARTESIAN_POINT('Origin',(2.9999999999999,35.9826602645987,63.0000000000002));
#13835=CARTESIAN_POINT('Origin',(380.64910337319,10.,25.0462333534358));
#13836=CARTESIAN_POINT('',(380.64910337319,3.,31.3962333534358));
#13837=CARTESIAN_POINT('Origin',(380.64910337319,3.,25.0462333534358));
#13838=CARTESIAN_POINT('',(380.64910337319,-4.44089209850063E-15,31.3962333534358));
#13839=CARTESIAN_POINT('',(380.64910337319,10.,31.3962333534358));
#13840=CARTESIAN_POINT('Origin',(380.64910337319,-3.06727895069828E-15,
25.0462333534358));
#13841=CARTESIAN_POINT('Origin',(304.66089662681,10.,25.0462333534316));
#13842=CARTESIAN_POINT('',(304.66089662681,3.,31.3962333534329));
#13843=CARTESIAN_POINT('Origin',(304.66089662681,3.,25.0462333534316));
#13844=CARTESIAN_POINT('',(304.66089662681,-4.44089209850063E-15,31.3962333534329));
#13845=CARTESIAN_POINT('',(304.66089662681,10.,31.3962333534329));
#13846=CARTESIAN_POINT('Origin',(304.66089662681,-3.06727895069777E-15,
25.0462333534316));
#13847=CARTESIAN_POINT('Origin',(342.655,9.99999999999997,213.158883372056));
#13848=CARTESIAN_POINT('',(342.655,3.,219.508883372057));
#13849=CARTESIAN_POINT('Origin',(342.655,3.,213.158883372056));
#13850=CARTESIAN_POINT('',(342.655,-2.77555756156289E-14,219.508883372057));
#13851=CARTESIAN_POINT('',(342.655,9.99999999999997,219.508883372057));
#13852=CARTESIAN_POINT('Origin',(342.655,-2.61044344231412E-14,213.158883372056));
#13853=CARTESIAN_POINT('Origin',(39.5,4.5,32.0000000000144));
#13854=CARTESIAN_POINT('',(39.5,3.,38.4629015223999));
#13855=CARTESIAN_POINT('Origin',(39.5,3.,32.0000000000144));
#13856=CARTESIAN_POINT('',(39.5,-5.55111512312578E-16,38.4629015223999));
#13857=CARTESIAN_POINT('',(39.5,4.5,38.4629015223999));
#13858=CARTESIAN_POINT('Origin',(39.5,0.,32.0000000000144));
#13859=CARTESIAN_POINT('Origin',(645.81,4.5,32.0000000000145));
#13860=CARTESIAN_POINT('',(645.81,3.,38.4629015224));
#13861=CARTESIAN_POINT('Origin',(645.81,3.,32.0000000000145));
#13862=CARTESIAN_POINT('',(645.81,0.,38.4629015224));
#13863=CARTESIAN_POINT('',(645.81,4.5,38.4629015224));
#13864=CARTESIAN_POINT('Origin',(645.81,0.,32.0000000000145));
#13865=CARTESIAN_POINT('Origin',(39.7099999999999,4.5,216.5));
#13866=CARTESIAN_POINT('',(39.7099999999999,3.,222.85));
#13867=CARTESIAN_POINT('Origin',(39.7099999999999,3.,216.5));
#13868=CARTESIAN_POINT('',(39.7099999999999,0.,222.85));
#13869=CARTESIAN_POINT('',(39.7099999999999,4.5,222.85));
#13870=CARTESIAN_POINT('Origin',(39.7099999999999,0.,216.5));
#13871=CARTESIAN_POINT('Origin',(645.6,4.5,216.5));
#13872=CARTESIAN_POINT('',(645.6,3.,222.85));
#13873=CARTESIAN_POINT('Origin',(645.6,3.,216.5));
#13874=CARTESIAN_POINT('',(645.6,0.,222.85));
#13875=CARTESIAN_POINT('',(645.6,4.5,222.85));
#13876=CARTESIAN_POINT('Origin',(645.6,0.,216.5));
#13877=CARTESIAN_POINT('Origin',(0.,66.,4.));
#13878=CARTESIAN_POINT('',(0.,66.,4.));
#13879=CARTESIAN_POINT('',(0.127016653792582,66.,4.));
#13880=CARTESIAN_POINT('',(0.,66.,4.));
#13881=CARTESIAN_POINT('',(4.,69.,4.));
#13882=CARTESIAN_POINT('Origin',(4.,65.,4.));
#13883=CARTESIAN_POINT('',(0.,69.,4.));
#13884=CARTESIAN_POINT('',(685.31,69.,3.99999999999926));
#13885=CARTESIAN_POINT('',(0.,69.,4.));
#13886=CARTESIAN_POINT('Origin',(4.,66.,175.030507120983));
#13887=CARTESIAN_POINT('',(4.,69.,175.030507120983));
#13888=CARTESIAN_POINT('',(0.,69.,175.030507120983));
#13889=CARTESIAN_POINT('',(685.31,69.,175.030507120983));
#13890=CARTESIAN_POINT('',(0.127016653792575,66.,175.030507120983));
#13891=CARTESIAN_POINT('Origin',(4.,65.,175.030507120983));
#13892=CARTESIAN_POINT('',(0.,66.,175.030507120983));
#13893=CARTESIAN_POINT('',(4.,66.,175.030507120983));
#13894=CARTESIAN_POINT('',(0.,66.,175.030507120983));
#13895=CARTESIAN_POINT('Origin',(685.31,69.,0.));
#13896=CARTESIAN_POINT('',(681.31,68.9999999999999,4.));
#13897=CARTESIAN_POINT('',(685.31,69.,4.));
#13898=CARTESIAN_POINT('',(4.,69.,3.99999999999999));
#13899=CARTESIAN_POINT('',(681.31,68.9999999999999,175.030507120983));
#13900=CARTESIAN_POINT('',(685.31,69.,175.030507120983));
#13901=CARTESIAN_POINT('',(681.31,68.9999999999999,175.030507120983));
#13902=CARTESIAN_POINT('Origin',(685.31,66.,-4.73106402539129E-16));
#13903=CARTESIAN_POINT('',(4.,66.,4.));
#13904=CARTESIAN_POINT('',(4.,66.,175.030507120983));
#13905=CARTESIAN_POINT('',(4.,66.,3.99999999999999));
#13906=CARTESIAN_POINT('',(681.31,66.,4.));
#13907=CARTESIAN_POINT('',(685.31,66.,4.));
#13908=CARTESIAN_POINT('',(681.31,65.9999999999999,175.030507120983));
#13909=CARTESIAN_POINT('',(681.31,65.9999999999999,175.030507120983));
#13910=CARTESIAN_POINT('',(685.31,66.,175.030507120983));
#13911=CARTESIAN_POINT('Origin',(685.31,66.,175.030507120983));
#13912=CARTESIAN_POINT('',(685.31,66.,175.030507120983));
#13913=CARTESIAN_POINT('',(685.182983346207,66.,175.030507120983));
#13914=CARTESIAN_POINT('',(685.31,66.,175.030507120983));
#13915=CARTESIAN_POINT('Origin',(681.31,64.9999999999999,175.030507120983));
#13916=CARTESIAN_POINT('',(685.31,69.,175.030507120983));
#13917=CARTESIAN_POINT('',(685.31,69.,175.030507120983));
#13918=CARTESIAN_POINT('',(685.31,69.,175.030507120983));
#13919=CARTESIAN_POINT('Origin',(681.31,65.9999999999999,4.));
#13920=CARTESIAN_POINT('',(685.31,69.,4.));
#13921=CARTESIAN_POINT('',(685.31,69.,4.));
#13922=CARTESIAN_POINT('',(685.182983346207,66.,4.));
#13923=CARTESIAN_POINT('Origin',(681.31,64.9999999999999,4.));
#13924=CARTESIAN_POINT('',(685.31,66.,4.));
#13925=CARTESIAN_POINT('',(685.31,66.,4.));
#13926=CARTESIAN_POINT('',(685.31,66.,4.));
#13927=CARTESIAN_POINT('Origin',(685.31,4.00000000000003,236.));
#13928=CARTESIAN_POINT('',(685.31,4.00000000000003,236.));
#13929=CARTESIAN_POINT('',(685.31,4.00000000000003,233.));
#13930=CARTESIAN_POINT('',(685.31,4.00000000000003,236.));
#13931=CARTESIAN_POINT('',(685.31,0.,232.));
#13932=CARTESIAN_POINT('Origin',(685.31,4.,232.));
#13933=CARTESIAN_POINT('',(685.31,3.,232.));
#13934=CARTESIAN_POINT('',(685.31,3.,232.));
#13935=CARTESIAN_POINT('Origin',(685.31,4.,232.));
#13936=CARTESIAN_POINT('Origin',(685.31,3.,232.));
#13937=CARTESIAN_POINT('',(685.31,35.6607111673065,236.));
#13938=CARTESIAN_POINT('',(685.31,38.1,236.));
#13939=CARTESIAN_POINT('',(685.31,35.6607111673065,233.));
#13940=CARTESIAN_POINT('',(685.31,38.1,233.));
#13941=CARTESIAN_POINT('',(685.31,35.6607111673065,233.));
#13942=CARTESIAN_POINT('Origin',(0.,0.,232.));
#13943=CARTESIAN_POINT('',(0.,0.,232.));
#13944=CARTESIAN_POINT('',(0.,3.,232.));
#13945=CARTESIAN_POINT('',(0.,0.,232.));
#13946=CARTESIAN_POINT('',(0.,4.00000000000003,236.));
#13947=CARTESIAN_POINT('Origin',(0.,4.,232.));
#13948=CARTESIAN_POINT('',(0.,4.00000000000003,233.));
#13949=CARTESIAN_POINT('',(0.,4.00000000000003,233.));
#13950=CARTESIAN_POINT('Origin',(0.,4.,232.));
#13951=CARTESIAN_POINT('Origin',(0.,4.00000000000003,233.));
#13952=CARTESIAN_POINT('',(0.,0.,201.));
#13953=CARTESIAN_POINT('',(0.,0.,236.));
#13954=CARTESIAN_POINT('',(0.,3.,201.));
#13955=CARTESIAN_POINT('',(0.,3.,236.));
#13956=CARTESIAN_POINT('',(0.,3.,201.));
#13957=CARTESIAN_POINT('Origin',(685.31,39.2168287216494,233.831400540487));
#13958=CARTESIAN_POINT('',(685.31,39.2168287216494,233.831400540487));
#13959=CARTESIAN_POINT('',(685.31,36.5497405558922,232.457850135122));
#13960=CARTESIAN_POINT('',(685.31,39.2168287216494,233.831400540487));
#13961=CARTESIAN_POINT('Origin',(685.31,35.6607111673065,232.));
#13962=CARTESIAN_POINT('Origin',(685.31,35.6607111673065,232.));
#13963=CARTESIAN_POINT('Origin',(685.31,35.6607111673065,233.));
#13964=CARTESIAN_POINT('',(685.31,68.5561175543429,176.86190766147));
#13965=CARTESIAN_POINT('',(685.31,69.,176.));
#13966=CARTESIAN_POINT('',(685.31,65.8890293885857,175.488357256105));
#13967=CARTESIAN_POINT('',(685.31,66.3329118342428,174.626449594635));
#13968=CARTESIAN_POINT('',(685.31,65.8890293885857,175.488357256105));
#13969=CARTESIAN_POINT('Origin',(0.,35.6607111673065,236.));
#13970=CARTESIAN_POINT('',(0.,35.6607111673065,236.));
#13971=CARTESIAN_POINT('',(0.,35.6607111673065,233.));
#13972=CARTESIAN_POINT('',(0.,35.6607111673065,236.));
#13973=CARTESIAN_POINT('',(0.,39.2168287216494,233.831400540487));
#13974=CARTESIAN_POINT('Origin',(0.,35.6607111673065,232.));
#13975=CARTESIAN_POINT('',(0.,36.5497405558922,232.457850135122));
#13976=CARTESIAN_POINT('',(0.,36.5497405558922,232.457850135122));
#13977=CARTESIAN_POINT('Origin',(0.,35.6607111673065,232.));
#13978=CARTESIAN_POINT('Origin',(0.,36.5497405558922,232.457850135122));
#13979=CARTESIAN_POINT('',(0.,38.1,236.));
#13980=CARTESIAN_POINT('',(0.,38.1,233.));
#13981=CARTESIAN_POINT('Origin',(685.31,69.,175.030507120983));
#13982=CARTESIAN_POINT('Origin',(685.31,65.,175.030507120983));
#13983=CARTESIAN_POINT('Origin',(685.31,65.,175.030507120983));
#13984=CARTESIAN_POINT('Origin',(0.,68.5561175543429,176.86190766147));
#13985=CARTESIAN_POINT('',(0.,68.5561175543429,176.86190766147));
#13986=CARTESIAN_POINT('',(0.,65.8890293885857,175.488357256105));
#13987=CARTESIAN_POINT('',(0.,68.5561175543429,176.86190766147));
#13988=CARTESIAN_POINT('Origin',(0.,65.,175.030507120983));
#13989=CARTESIAN_POINT('Origin',(0.,65.,175.030507120983));
#13990=CARTESIAN_POINT('Origin',(0.,66.,175.030507120983));
#13991=CARTESIAN_POINT('',(0.,69.,176.));
#13992=CARTESIAN_POINT('',(0.,66.3329118342428,174.626449594635));
#13993=CARTESIAN_POINT('Origin',(685.31,65.,0.));
#13994=CARTESIAN_POINT('',(685.31,65.,0.));
#13995=CARTESIAN_POINT('',(685.31,65.,3.));
#13996=CARTESIAN_POINT('',(685.31,65.,0.));
#13997=CARTESIAN_POINT('Origin',(685.31,65.,4.));
#13998=CARTESIAN_POINT('Origin',(685.31,65.,4.));
#13999=CARTESIAN_POINT('Origin',(685.31,66.,4.));
#14000=CARTESIAN_POINT('',(685.31,4.,0.));
#14001=CARTESIAN_POINT('',(685.31,0.,0.));
#14002=CARTESIAN_POINT('',(685.31,4.,3.));
#14003=CARTESIAN_POINT('',(685.31,0.,3.));
#14004=CARTESIAN_POINT('',(685.31,4.,3.));
#14005=CARTESIAN_POINT('Origin',(0.,69.,4.));
#14006=CARTESIAN_POINT('',(0.,65.,0.));
#14007=CARTESIAN_POINT('Origin',(0.,65.,4.));
#14008=CARTESIAN_POINT('',(0.,65.,3.));
#14009=CARTESIAN_POINT('',(0.,65.,3.));
#14010=CARTESIAN_POINT('Origin',(0.,65.,4.));
#14011=CARTESIAN_POINT('Origin',(685.31,-4.89858719658941E-16,4.));
#14012=CARTESIAN_POINT('',(685.31,-4.89858719658941E-16,4.));
#14013=CARTESIAN_POINT('',(685.31,3.,4.));
#14014=CARTESIAN_POINT('',(685.31,-4.89858719658941E-16,4.));
#14015=CARTESIAN_POINT('Origin',(685.31,4.,4.));
#14016=CARTESIAN_POINT('Origin',(685.31,4.,4.));
#14017=CARTESIAN_POINT('Origin',(685.31,4.,3.));
#14018=CARTESIAN_POINT('',(685.31,-7.47034547479886E-15,61.));
#14019=CARTESIAN_POINT('',(685.31,0.,0.));
#14020=CARTESIAN_POINT('',(685.31,2.99999999999999,61.));
#14021=CARTESIAN_POINT('',(685.31,3.,3.67394039744206E-16));
#14022=CARTESIAN_POINT('',(685.31,-7.47034547479886E-15,61.));
#14023=CARTESIAN_POINT('Origin',(0.,4.,0.));
#14024=CARTESIAN_POINT('',(0.,4.,0.));
#14025=CARTESIAN_POINT('',(0.,4.,3.));
#14026=CARTESIAN_POINT('',(0.,4.,0.));
#14027=CARTESIAN_POINT('',(0.,-4.89858719658941E-16,4.));
#14028=CARTESIAN_POINT('Origin',(0.,4.,4.));
#14029=CARTESIAN_POINT('',(0.,3.,4.));
#14030=CARTESIAN_POINT('',(0.,3.,4.));
#14031=CARTESIAN_POINT('Origin',(0.,4.,4.));
#14032=CARTESIAN_POINT('Origin',(0.,3.,4.));
#14033=CARTESIAN_POINT('',(0.,0.,0.));
#14034=CARTESIAN_POINT('',(0.,0.,3.));
#14035=CARTESIAN_POINT('Origin',(685.31,3.,3.67394039744206E-16));
#14036=CARTESIAN_POINT('',(0.,2.99999999999999,61.));
#14037=CARTESIAN_POINT('',(0.,3.,3.67394039744206E-16));
#14038=CARTESIAN_POINT('',(685.31,2.99999999999999,61.));
#14039=CARTESIAN_POINT('',(685.31,3.,4.));
#14040=CARTESIAN_POINT('Origin',(685.31,-7.47034547479886E-15,61.));
#14041=CARTESIAN_POINT('',(0.,-7.47034547479886E-15,61.));
#14042=CARTESIAN_POINT('',(0.,-7.47034547479886E-15,61.));
#14043=CARTESIAN_POINT('',(685.31,-7.47034547479886E-15,61.));
#14044=CARTESIAN_POINT('Origin',(685.31,0.,0.));
#14045=CARTESIAN_POINT('',(0.,0.,0.));
#14046=CARTESIAN_POINT('',(685.31,-4.89858719658941E-16,4.));
#14047=CARTESIAN_POINT('Origin',(685.31,4.,4.));
#14048=CARTESIAN_POINT('',(685.31,4.,0.));
#14049=CARTESIAN_POINT('Origin',(685.31,0.,0.));
#14050=CARTESIAN_POINT('',(685.31,65.,0.));
#14051=CARTESIAN_POINT('Origin',(685.31,65.,4.));
#14052=CARTESIAN_POINT('Origin',(685.31,65.,175.030507120983));
#14053=CARTESIAN_POINT('',(685.31,68.5561175543429,176.86190766147));
#14054=CARTESIAN_POINT('Origin',(685.31,69.,176.));
#14055=CARTESIAN_POINT('',(685.31,39.2168287216494,233.831400540487));
#14056=CARTESIAN_POINT('Origin',(685.31,35.6607111673065,232.));
#14057=CARTESIAN_POINT('',(685.31,35.6607111673065,236.));
#14058=CARTESIAN_POINT('Origin',(685.31,38.1,236.));
#14059=CARTESIAN_POINT('',(685.31,4.00000000000003,236.));
#14060=CARTESIAN_POINT('Origin',(685.31,4.,232.));
#14061=CARTESIAN_POINT('',(685.31,0.,232.));
#14062=CARTESIAN_POINT('Origin',(685.31,0.,236.));
#14063=CARTESIAN_POINT('',(685.31,0.,201.));
#14064=CARTESIAN_POINT('',(685.31,0.,201.));
#14065=CARTESIAN_POINT('',(685.31,0.,236.));
#14066=CARTESIAN_POINT('Origin',(685.31,3.,201.));
#14067=CARTESIAN_POINT('',(685.31,3.,201.));
#14068=CARTESIAN_POINT('',(685.31,3.,201.));
#14069=CARTESIAN_POINT('',(685.31,3.,201.));
#14070=CARTESIAN_POINT('Origin',(685.31,3.,236.));
#14071=CARTESIAN_POINT('',(685.31,3.,232.));
#14072=CARTESIAN_POINT('',(685.31,3.,236.));
#14073=CARTESIAN_POINT('Origin',(685.31,4.,232.));
#14074=CARTESIAN_POINT('',(685.31,4.00000000000003,233.));
#14075=CARTESIAN_POINT('Origin',(685.31,38.1,233.));
#14076=CARTESIAN_POINT('',(685.31,35.6607111673065,233.));
#14077=CARTESIAN_POINT('Origin',(685.31,35.6607111673065,232.));
#14078=CARTESIAN_POINT('',(685.31,36.5497405558922,232.457850135122));
#14079=CARTESIAN_POINT('Origin',(685.31,66.3329118342428,174.626449594635));
#14080=CARTESIAN_POINT('',(685.31,65.8890293885857,175.488357256105));
#14081=CARTESIAN_POINT('Origin',(685.31,65.,175.030507120983));
#14082=CARTESIAN_POINT('',(4.,66.,175.030507120983));
#14083=CARTESIAN_POINT('',(685.31,66.,175.030507120983));
#14084=CARTESIAN_POINT('Origin',(685.31,65.,4.));
#14085=CARTESIAN_POINT('',(685.31,65.,3.));
#14086=CARTESIAN_POINT('',(685.31,66.,4.));
#14087=CARTESIAN_POINT('',(0.,66.,4.));
#14088=CARTESIAN_POINT('Origin',(685.31,0.,3.));
#14089=CARTESIAN_POINT('',(685.31,4.,3.));
#14090=CARTESIAN_POINT('Origin',(685.31,4.,4.));
#14091=CARTESIAN_POINT('Origin',(685.31,4.,4.));
#14092=CARTESIAN_POINT('Origin',(0.,4.,4.));
#14093=CARTESIAN_POINT('Origin',(681.31,64.9999999999999,4.));
#14094=CARTESIAN_POINT('',(685.31,64.9999999999999,4.));
#14095=CARTESIAN_POINT('Origin',(681.31,64.9999999999999,4.));
#14096=CARTESIAN_POINT('',(682.31,64.9999999999999,4.));
#14097=CARTESIAN_POINT('',(685.31,65.,4.));
#14098=CARTESIAN_POINT('Origin',(681.31,64.9999999999999,4.));
#14099=CARTESIAN_POINT('Origin',(681.31,64.9999999999999,175.030507120983));
#14100=CARTESIAN_POINT('',(685.31,65.,175.030507120983));
#14101=CARTESIAN_POINT('Origin',(681.31,64.9999999999999,175.030507120983));
#14102=CARTESIAN_POINT('',(682.31,64.9999999999999,175.030507120983));
#14103=CARTESIAN_POINT('Origin',(681.31,64.9999999999999,175.030507120983));
#14104=CARTESIAN_POINT('',(682.31,64.9999999999999,175.030507120983));
#14105=CARTESIAN_POINT('Origin',(681.31,64.9999999999999,175.030507120983));
#14106=CARTESIAN_POINT('',(685.31,65.,3.99999999999999));
#14107=CARTESIAN_POINT('Origin',(681.31,64.9999999999999,175.030507120983));
#14108=CARTESIAN_POINT('',(682.31,64.9999999999999,3.99999999999999));
#14109=CARTESIAN_POINT('Origin',(685.31,8.99999999999998,175.030507120983));
#14110=CARTESIAN_POINT('',(682.31,62.0111994331027,175.030507120983));
#14111=CARTESIAN_POINT('',(682.31,8.99999999999996,175.030507120983));
#14112=CARTESIAN_POINT('',(685.31,62.0111994331027,175.030507120983));
#14113=CARTESIAN_POINT('',(682.31,62.0111994331027,175.030507120983));
#14114=CARTESIAN_POINT('',(685.31,2.6801128335108E-12,175.030507120983));
#14115=CARTESIAN_POINT('Origin',(685.31,66.,4.));
#14116=CARTESIAN_POINT('',(685.31,9.00000000000001,3.99999999999999));
#14117=CARTESIAN_POINT('',(685.31,2.67932155613579E-12,3.99999999999999));
#14118=CARTESIAN_POINT('',(682.31,8.99999999999999,3.99999999999999));
#14119=CARTESIAN_POINT('',(685.31,9.00000000000001,3.99999999999999));
#14120=CARTESIAN_POINT('',(682.31,66.,4.));
#14121=CARTESIAN_POINT('Origin',(685.31,2.6801128335108E-12,4.3494038380127E-28));
#14122=CARTESIAN_POINT('',(685.31,34.9708140306692,228.641008611614));
#14123=CARTESIAN_POINT('',(685.31,62.0111994331027,175.030507120983));
#14124=CARTESIAN_POINT('',(685.31,8.99999999999998,228.641008611614));
#14125=CARTESIAN_POINT('',(685.31,34.9708140306692,228.641008611614));
#14126=CARTESIAN_POINT('',(685.31,9.00000000000001,1.46055919932435E-15));
#14127=CARTESIAN_POINT('Origin',(682.31,2.66963838949427E-12,4.33240545405031E-28));
#14128=CARTESIAN_POINT('',(682.31,8.99999999999997,228.641008611614));
#14129=CARTESIAN_POINT('',(682.31,8.99999999999999,3.99999999999999));
#14130=CARTESIAN_POINT('',(682.31,34.9708140306692,228.641008611614));
#14131=CARTESIAN_POINT('',(682.31,34.9708140306692,228.641008611614));
#14132=CARTESIAN_POINT('',(682.31,62.0111994331027,175.030507120983));
#14133=CARTESIAN_POINT('Origin',(685.31,9.00000000000001,3.99999999999999));
#14134=CARTESIAN_POINT('',(682.31,8.99999999999997,228.641008611614));
#14135=CARTESIAN_POINT('Origin',(682.31,34.9708140306692,228.641008611614));
#14136=CARTESIAN_POINT('',(682.31,34.9708140306692,228.641008611614));
#14137=CARTESIAN_POINT('Origin',(682.31,62.0111994331027,175.030507120983));
#14138=CARTESIAN_POINT('Origin',(4.,65.,175.030507120983));
#14139=CARTESIAN_POINT('',(3.,65.,175.030507120983));
#14140=CARTESIAN_POINT('Origin',(4.,65.,175.030507120983));
#14141=CARTESIAN_POINT('',(-1.73472347597681E-15,65.,175.030507120983));
#14142=CARTESIAN_POINT('Origin',(4.,65.,175.030507120983));
#14143=CARTESIAN_POINT('',(-3.4914813388431E-15,65.,175.030507120983));
#14144=CARTESIAN_POINT('Origin',(4.,65.,4.));
#14145=CARTESIAN_POINT('',(-3.43664881674456E-15,65.,4.));
#14146=CARTESIAN_POINT('Origin',(4.,65.,4.));
#14147=CARTESIAN_POINT('',(3.,65.,4.));
#14148=CARTESIAN_POINT('Origin',(4.,65.,4.));
#14149=CARTESIAN_POINT('',(3.,65.,4.));
#14150=CARTESIAN_POINT('Origin',(4.,65.,3.99999999999999));
#14151=CARTESIAN_POINT('',(-3.46944695195361E-15,65.,175.030507120983));
#14152=CARTESIAN_POINT('Origin',(4.,65.,3.99999999999999));
#14153=CARTESIAN_POINT('',(3.,65.,175.030507120983));
#14154=CARTESIAN_POINT('Origin',(0.,66.,175.030507120983));
#14155=CARTESIAN_POINT('',(-1.37735958159548E-14,62.0111994331051,175.030507120983));
#14156=CARTESIAN_POINT('',(-2.30284541435921E-13,1.04744440165302E-14,175.030507120983));
#14157=CARTESIAN_POINT('',(2.99999999999999,62.0111994331051,175.030507120983));
#14158=CARTESIAN_POINT('',(3.00000000000022,62.0111994331051,175.030507120983));
#14159=CARTESIAN_POINT('',(3.,66.,175.030507120983));
#14160=CARTESIAN_POINT('Origin',(-1.99059518868339E-13,9.00000000000001,
3.99999999999998));
#14161=CARTESIAN_POINT('',(2.9999999999998,8.99999999999999,3.99999999999998));
#14162=CARTESIAN_POINT('',(2.9999999999998,8.99999999999999,3.99999999999998));
#14163=CARTESIAN_POINT('',(-1.98861209386333E-13,9.00000000000001,3.99999999999998));
#14164=CARTESIAN_POINT('',(-1.99059518868339E-13,9.00000000000001,3.99999999999998));
#14165=CARTESIAN_POINT('',(-2.30284541435921E-13,8.95275675690144E-15,3.99999999999998));
#14166=CARTESIAN_POINT('Origin',(-2.30284541435921E-13,1.04744440165302E-14,
1.699838396239E-30));
#14167=CARTESIAN_POINT('',(3.14233320495966E-14,9.00000000000237,228.641008611614));
#14168=CARTESIAN_POINT('',(-1.98861209386333E-13,9.00000000000001,1.46055919932435E-15));
#14169=CARTESIAN_POINT('',(1.22099944592244E-13,34.9708140306716,228.641008611614));
#14170=CARTESIAN_POINT('',(3.14233320495966E-14,9.00000000000237,228.641008611614));
#14171=CARTESIAN_POINT('',(1.22099944592244E-13,34.9708140306716,228.641008611614));
#14172=CARTESIAN_POINT('Origin',(2.99999999999977,8.04569168006329E-28,
1.30568988869375E-43));
#14173=CARTESIAN_POINT('',(3.00000000000012,34.9708140306716,228.641008611614));
#14174=CARTESIAN_POINT('',(3.00000000000012,34.9708140306716,228.641008611614));
#14175=CARTESIAN_POINT('',(3.00000000000003,9.00000000000236,228.641008611614));
#14176=CARTESIAN_POINT('',(3.00000000000003,9.00000000000236,228.641008611614));
#14177=CARTESIAN_POINT('',(2.9999999999998,8.99999999999997,175.030507120983));
#14178=CARTESIAN_POINT('Origin',(-1.99059518868339E-13,8.99999999999998,
175.030507120983));
#14179=CARTESIAN_POINT('',(3.00000000000003,9.00000000000236,228.641008611614));
#14180=CARTESIAN_POINT('Origin',(3.00000000000012,34.9708140306716,228.641008611614));
#14181=CARTESIAN_POINT('',(3.00000000000012,34.9708140306716,228.641008611614));
#14182=CARTESIAN_POINT('Origin',(3.00000000000003,9.00000000000236,228.641008611614));
#17968=UNCERTAINTY_MEASURE_WITH_UNIT(LENGTH_MEASURE(0.01),#18007,
'DISTANCE_ACCURACY_VALUE',
'Maximum model space distance between geometric entities at asserted c
onnectivities');
#17986=UNCERTAINTY_MEASURE_WITH_UNIT(LENGTH_MEASURE(0.01),#18007,
'DISTANCE_ACCURACY_VALUE',
'Maximum model space distance between geometric entities at asserted c
onnectivities');
#17988=(
GEOMETRIC_REPRESENTATION_CONTEXT(3)
GLOBAL_UNCERTAINTY_ASSIGNED_CONTEXT((#17968))
GLOBAL_UNIT_ASSIGNED_CONTEXT((#18007,#18009,#18010))
REPRESENTATION_CONTEXT('','3D')
);
#18006=(
GEOMETRIC_REPRESENTATION_CONTEXT(3)
GLOBAL_UNCERTAINTY_ASSIGNED_CONTEXT((#17986))
GLOBAL_UNIT_ASSIGNED_CONTEXT((#18007,#18009,#18010))
REPRESENTATION_CONTEXT('','3D')
);
#18007=(
LENGTH_UNIT()
NAMED_UNIT(*)
SI_UNIT(.MILLI.,.METRE.)
);
#18009=(
NAMED_UNIT(*)
PLANE_ANGLE_UNIT()
SI_UNIT($,.RADIAN.)
);
#18010=(
NAMED_UNIT(*)
SI_UNIT($,.STERADIAN.)
SOLID_ANGLE_UNIT()
);
#18012=SHAPE_DEFINITION_REPRESENTATION(#18031,#18071);
#18031=PRODUCT_DEFINITION_SHAPE('',$,#18091);
#18071=SHAPE_REPRESENTATION('',(#9750),#17988);
#18089=PRODUCT_DEFINITION_CONTEXT('part definition',#18148,'design');
#18091=PRODUCT_DEFINITION('Bottom Rail','Bottom Rail',#18110,#18089);
#18110=PRODUCT_DEFINITION_FORMATION('',$,#18151);
#18148=APPLICATION_CONTEXT(
'Core Data for Automotive Mechanical Design Process');
#18149=PRODUCT_CONTEXT('part definition',#18148,'mechanical');
#18151=PRODUCT('Bottom Rail','Bottom Rail',$,(#18149));
#18170=PRESENTATION_STYLE_ASSIGNMENT((#18174));
#18174=SURFACE_STYLE_USAGE(.BOTH.,#18178);
#18178=SURFACE_SIDE_STYLE('',(#18182));
#18182=SURFACE_STYLE_FILL_AREA(#18186);
#18186=FILL_AREA_STYLE('Opaque(227,224,212)',(#18190));
#18190=FILL_AREA_STYLE_COLOUR('Opaque(227,224,212)',#18194);
#18194=COLOUR_RGB('Opaque(227,224,212)',0.890196078431372,0.87843137254902,
0.831372549019608);
ENDSEC;
END-ISO-10303-21;
